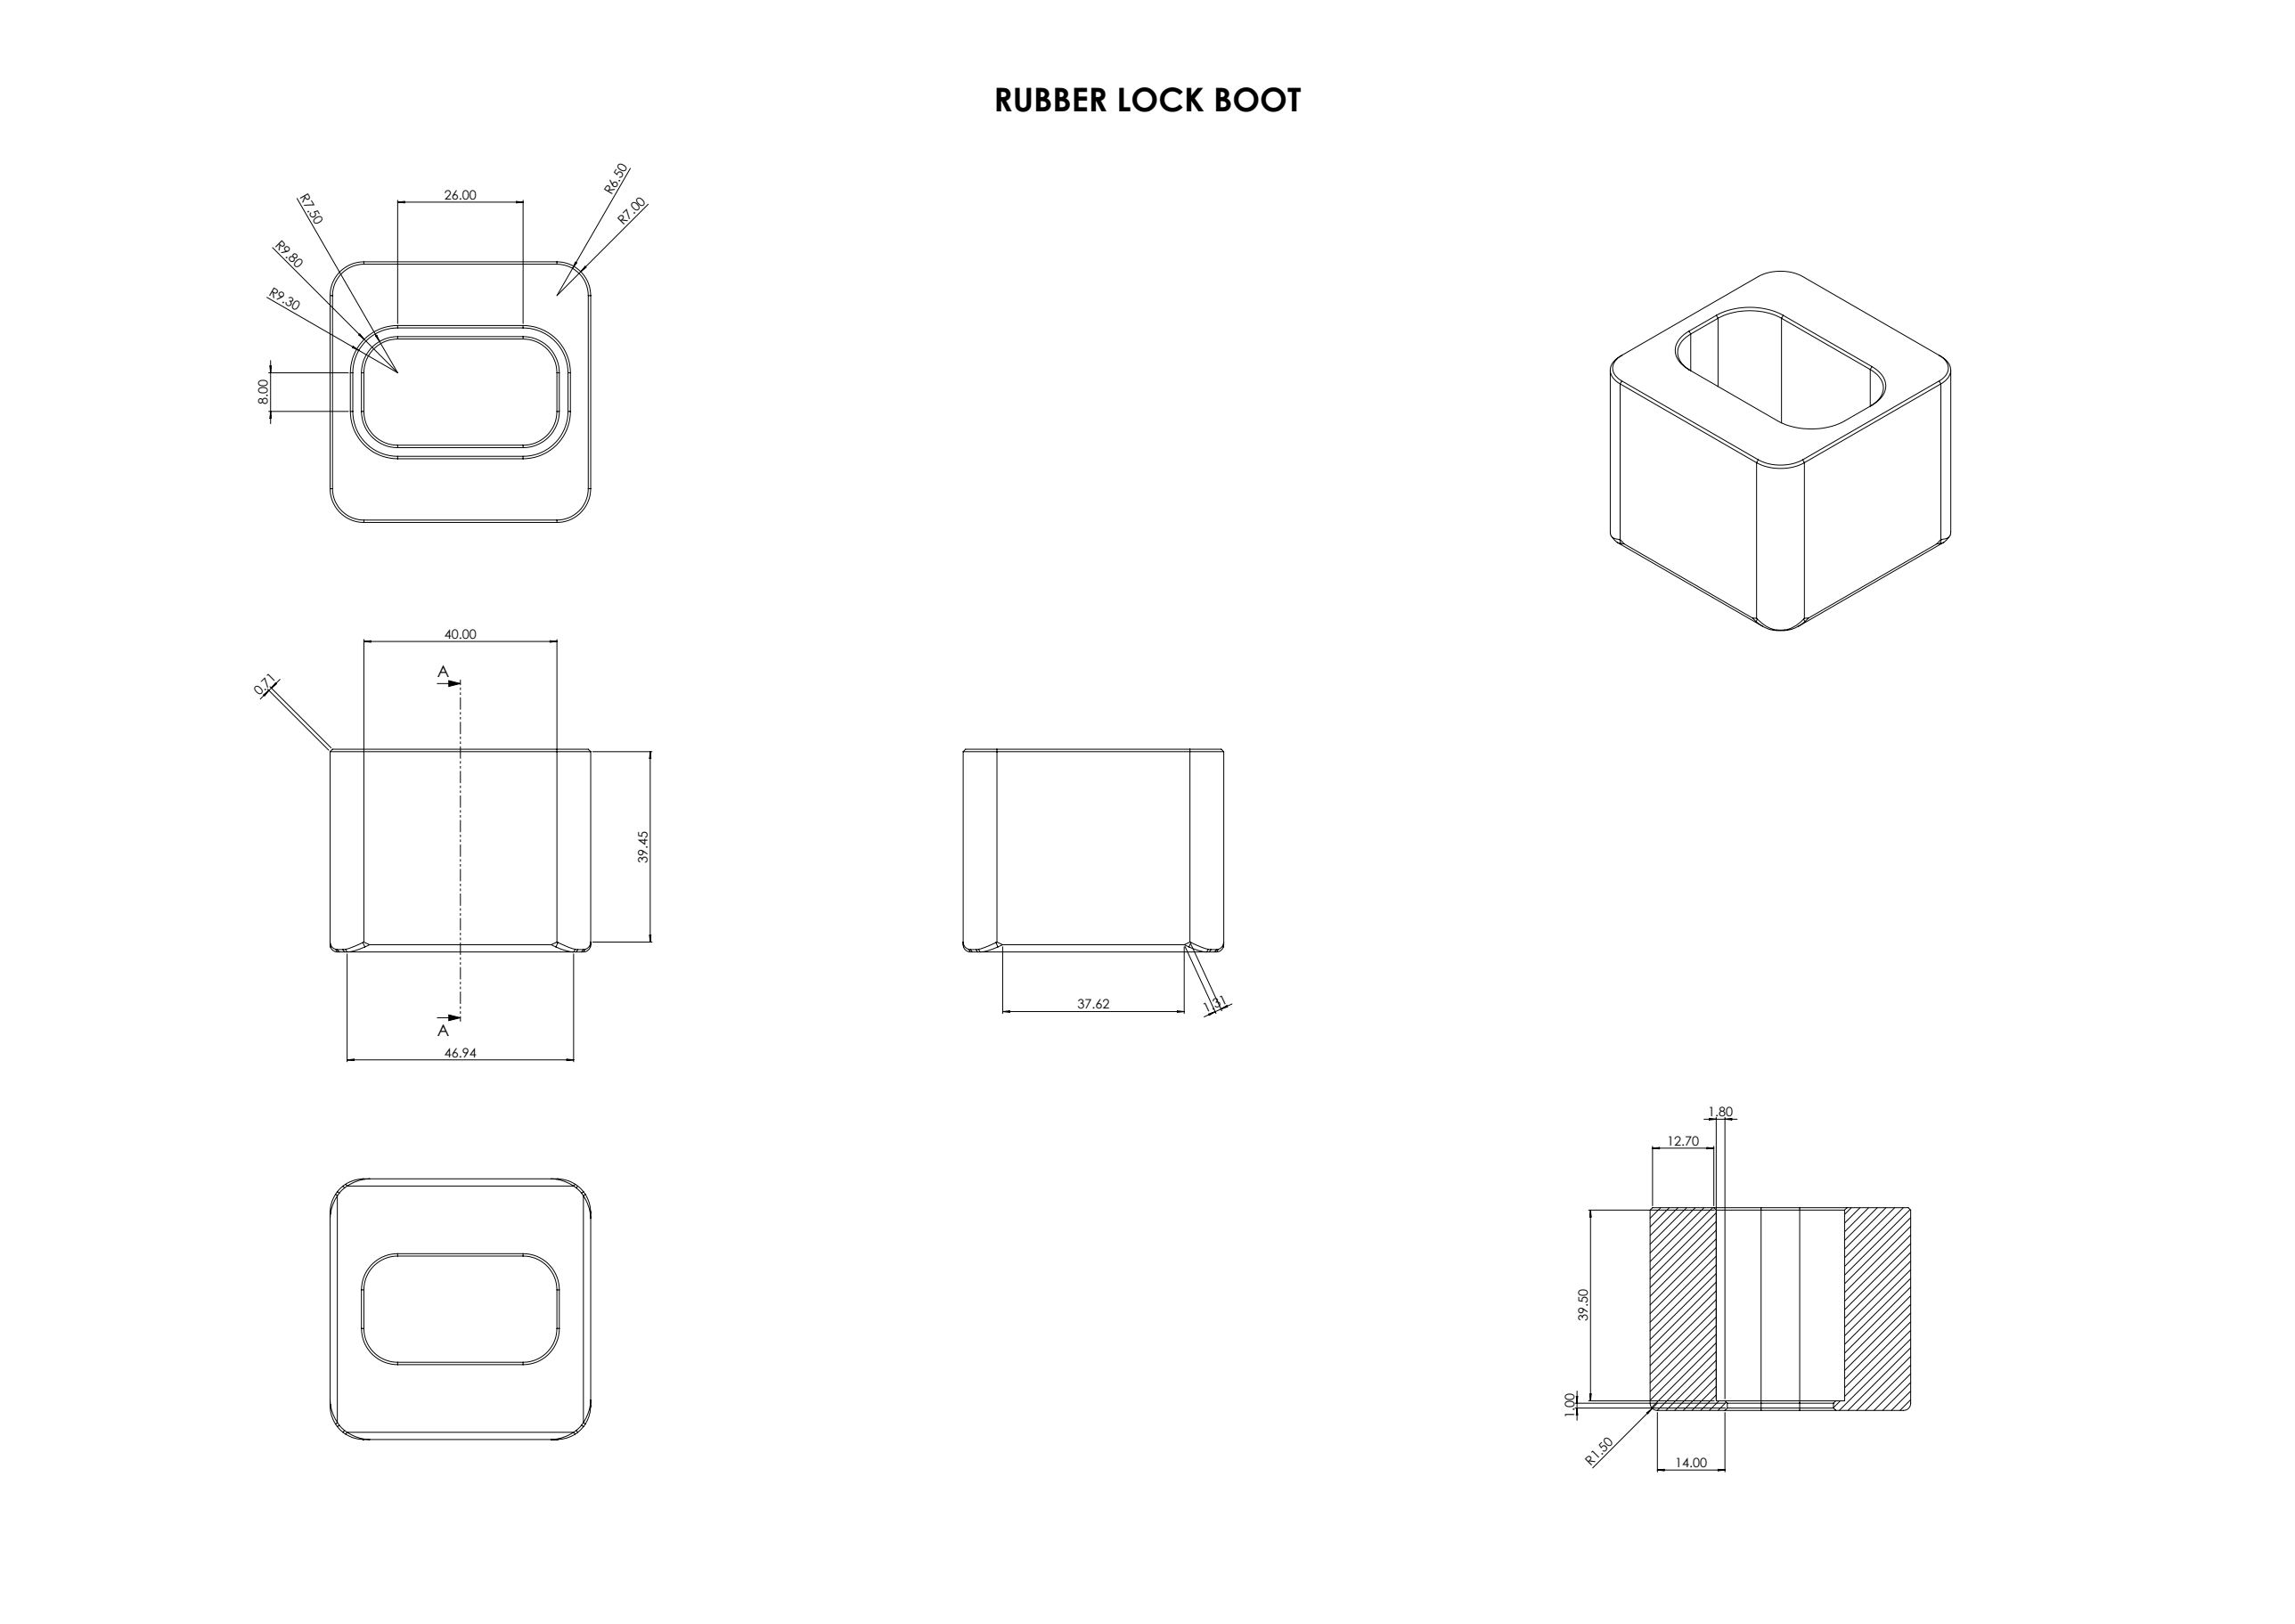
ISO-10303-21;
HEADER;
/* Generated by software containing ST-Developer
 * from STEP Tools, Inc. (www.steptools.com) 
 */

FILE_DESCRIPTION(
/* description */ (''),
/* implementation_level */ '2;1');

FILE_NAME(
/* name */ '13_Rubber_Lock_Boot.step',
/* time_stamp */ '2026-10-25T01:30:15-07:00',
/* author */ (''),
/* organization */ (''),
/* preprocessor_version */ 'ST-DEVELOPER v20.2',
/* originating_system */ 'Autodesk Translation Framework v15.15.0.0',
/* authorisation */ '');

FILE_SCHEMA (('AUTOMOTIVE_DESIGN { 1 0 10303 214 3 1 1 }'));
ENDSEC;

DATA;
#10=MECHANICAL_DESIGN_GEOMETRIC_PRESENTATION_REPRESENTATION('',(#574),#32309);
#296=B_SPLINE_CURVE_WITH_KNOTS('',3,(#27048,#27049,#27050,#27051,#27052,
#27053,#27054,#27055,#27056,#27057,#27058,#27059,#27060,#27061,#27062,#27063,
#27064,#27065,#27066,#27067,#27068,#27069,#27070,#27071,#27072,#27073,#27074,
#27075,#27076,#27077,#27078,#27079,#27080,#27081,#27082,#27083,#27084,#27085,
#27086,#27087,#27088,#27089,#27090,#27091,#27092,#27093,#27094,#27095,#27096,
#27097,#27098,#27099,#27100,#27101,#27102,#27103,#27104,#27105,#27106,#27107,
#27108,#27109,#27110,#27111,#27112,#27113,#27114),.UNSPECIFIED.,.F.,.F.,
(4,3,3,3,3,3,3,3,3,3,3,3,3,3,3,3,3,3,3,3,3,3,4),(0.,0.0372150073459974,
0.0759036440357819,0.116494755002558,0.15971628635105,0.207036887347821,
0.265275351739583,0.328858620274534,0.377066398240659,0.420570421282261,
0.461281571881092,0.50247045159648,0.542638283169258,0.585163636770142,
0.631190064016801,0.685017456026248,0.763763092019686,0.814055107507527,
0.860541330630645,0.901120921336454,0.940124312769201,0.977290078168108,
1.),.UNSPECIFIED.);
#297=B_SPLINE_CURVE_WITH_KNOTS('',3,(#27116,#27117,#27118,#27119,#27120),
 .UNSPECIFIED.,.F.,.F.,(4,1,4),(1.09621611801068,1.29877304187851,1.50132996574633),
 .UNSPECIFIED.);
#298=B_SPLINE_CURVE_WITH_KNOTS('',3,(#27122,#27123,#27124,#27125),
 .UNSPECIFIED.,.F.,.F.,(4,4),(1.02439235355261,1.09621611801068),
 .UNSPECIFIED.);
#299=B_SPLINE_CURVE_WITH_KNOTS('',3,(#27129,#27130,#27131,#27132),
 .UNSPECIFIED.,.F.,.F.,(4,4),(0.396818713712603,0.466059241584687),
 .UNSPECIFIED.);
#300=B_SPLINE_CURVE_WITH_KNOTS('',3,(#27134,#27135,#27136,#27137,#27138,
#27139,#27140),.UNSPECIFIED.,.F.,.F.,(4,2,1,4),(9.99213751786565E-5,0.127637384843918,
0.289146182165162,0.396818713712658),.UNSPECIFIED.);
#301=B_SPLINE_CURVE_WITH_KNOTS('',3,(#27141,#27142,#27143,#27144,#27145,
#27146,#27147,#27148,#27149,#27150,#27151,#27152,#27153,#27154,#27155,#27156,
#27157,#27158,#27159,#27160,#27161,#27162,#27163,#27164,#27165,#27166,#27167,
#27168,#27169,#27170,#27171,#27172,#27173,#27174,#27175,#27176,#27177,#27178,
#27179,#27180,#27181,#27182,#27183,#27184,#27185,#27186,#27187,#27188,#27189,
#27190,#27191,#27192,#27193,#27194,#27195,#27196,#27197,#27198,#27199,#27200,
#27201,#27202,#27203,#27204,#27205,#27206,#27207),.UNSPECIFIED.,.F.,.F.,
(4,3,3,3,3,3,3,3,3,3,3,3,3,3,3,3,3,3,3,3,3,3,4),(0.,0.0372142743249414,
0.0759021060272706,0.116492303751609,0.15971273797737,0.207031854381263,
0.265265992983546,0.328853755149798,0.37706150936917,0.420565256169277,
0.461276052626863,0.50245372219686,0.542621232263039,0.585145966617605,
0.631171144882026,0.684995344588453,0.76374650844134,0.814042029226479,
0.860531521919859,0.901112266515804,0.94011665297404,0.977283203644708,
1.),.UNSPECIFIED.);
#302=B_SPLINE_CURVE_WITH_KNOTS('',3,(#27220,#27221,#27222,#27223,#27224,
#27225,#27226,#27227,#27228,#27229,#27230,#27231,#27232,#27233,#27234,#27235,
#27236,#27237,#27238,#27239,#27240,#27241,#27242,#27243,#27244,#27245,#27246,
#27247,#27248,#27249,#27250,#27251,#27252,#27253,#27254,#27255,#27256,#27257,
#27258,#27259,#27260,#27261,#27262,#27263,#27264,#27265,#27266,#27267,#27268,
#27269,#27270,#27271,#27272,#27273,#27274,#27275,#27276,#27277,#27278,#27279,
#27280,#27281,#27282,#27283,#27284,#27285,#27286),.UNSPECIFIED.,.F.,.F.,
(4,3,3,3,3,3,3,3,3,3,3,3,3,3,3,3,3,3,3,3,3,3,4),(0.,0.0372150196070085,
0.0759036698970674,0.116494796498611,0.15971634697478,0.207036974548953,
0.265275520854355,0.328858695194123,0.377066470534805,0.420570496312742,
0.461281651387635,0.502470683175898,0.542638526520072,0.585163896376155,
0.631190349090315,0.685017798075316,0.763763348556487,0.814055329762754,
0.860541497322065,0.901121082418717,0.94012446955152,0.977290233255848,
1.),.UNSPECIFIED.);
#303=B_SPLINE_CURVE_WITH_KNOTS('',3,(#27288,#27289,#27290,#27291,#27292,
#27293),.UNSPECIFIED.,.F.,.F.,(4,1,1,4),(1.09363288142463,1.20698114379938,
1.26365527498675,1.49035179973623),.UNSPECIFIED.);
#304=B_SPLINE_CURVE_WITH_KNOTS('',3,(#27295,#27296,#27297,#27298),
 .UNSPECIFIED.,.F.,.F.,(4,4),(1.02439235355261,1.09363288142469),
 .UNSPECIFIED.);
#305=B_SPLINE_CURVE_WITH_KNOTS('',3,(#27302,#27303,#27304,#27305),
 .UNSPECIFIED.,.F.,.F.,(4,4),(0.405213665159311,0.477037429617386),
 .UNSPECIFIED.);
#306=B_SPLINE_CURVE_WITH_KNOTS('',3,(#27307,#27308,#27309,#27310,#27311),
 .UNSPECIFIED.,.F.,.F.,(4,1,4),(0.000100096646392837,0.202656880902853,
0.405213665159313),.UNSPECIFIED.);
#307=B_SPLINE_CURVE_WITH_KNOTS('',3,(#27312,#27313,#27314,#27315,#27316,
#27317,#27318,#27319,#27320,#27321,#27322,#27323,#27324,#27325,#27326,#27327,
#27328,#27329,#27330,#27331,#27332,#27333,#27334,#27335,#27336,#27337,#27338,
#27339,#27340,#27341,#27342,#27343,#27344,#27345,#27346,#27347,#27348,#27349,
#27350,#27351,#27352,#27353,#27354,#27355,#27356,#27357,#27358,#27359,#27360,
#27361,#27362,#27363,#27364,#27365,#27366,#27367,#27368,#27369,#27370,#27371,
#27372,#27373,#27374,#27375,#27376,#27377,#27378),.UNSPECIFIED.,.F.,.F.,
(4,3,3,3,3,3,3,3,3,3,3,3,3,3,3,3,3,3,3,3,3,3,4),(0.,0.0372142122738283,
0.0759019766651123,0.116492099285913,0.159712445400096,0.207031446837133,
0.265265278177762,0.328853304622193,0.377061038248202,0.420564750072856,
0.461275507649365,0.502452205884434,0.542619564376986,0.585144107738491,
0.631169015934125,0.684992668379561,0.763744501284671,0.81404021150862,
0.860530158631465,0.901110881237409,0.94011523948485,0.977281743245876,
1.),.UNSPECIFIED.);
#308=B_SPLINE_CURVE_WITH_KNOTS('',3,(#27420,#27421,#27422,#27423,#27424,
#27425,#27426,#27427,#27428,#27429,#27430,#27431,#27432,#27433,#27434,#27435,
#27436,#27437,#27438,#27439,#27440,#27441,#27442,#27443,#27444,#27445,#27446,
#27447,#27448,#27449,#27450,#27451,#27452,#27453,#27454,#27455,#27456,#27457,
#27458,#27459,#27460,#27461,#27462,#27463,#27464,#27465,#27466,#27467,#27468,
#27469,#27470,#27471,#27472,#27473,#27474,#27475,#27476,#27477,#27478,#27479,
#27480,#27481,#27482,#27483,#27484,#27485,#27486,#27487,#27488,#27489,#27490,
#27491,#27492,#27493,#27494,#27495,#27496,#27497,#27498,#27499,#27500,#27501,
#27502,#27503,#27504,#27505,#27506,#27507,#27508,#27509,#27510,#27511,#27512,
#27513,#27514,#27515,#27516),.UNSPECIFIED.,.F.,.F.,(4,3,3,3,3,3,3,3,3,3,
3,3,3,3,3,3,3,3,3,3,3,3,3,3,3,3,3,3,3,3,3,3,4),(0.,0.0249561576389582,0.0505230689649538,
0.0768014946929841,0.103927702815189,0.132729761515055,0.163050828032849,
0.195526914275497,0.231526666456084,0.275596223262613,0.320871459308699,
0.357021183774404,0.38928558844534,0.419345587098888,0.447888984260675,
0.475288232374118,0.503212894511638,0.530052590323374,0.557847043091744,
0.587565866489206,0.619084976767266,0.653310159114776,0.692899272183232,
0.744530806263077,0.780991793284318,0.81370690045686,0.84424865112698,0.87328209994709,
0.901172514215133,0.927739555510914,0.953706026754902,0.978856478652302,
1.),.UNSPECIFIED.);
#309=B_SPLINE_CURVE_WITH_KNOTS('',3,(#27518,#27519,#27520,#27521),
 .UNSPECIFIED.,.F.,.F.,(4,4),(-1.,0.),.UNSPECIFIED.);
#310=B_SPLINE_CURVE_WITH_KNOTS('',3,(#27522,#27523,#27524,#27525,#27526,
#27527,#27528,#27529,#27530,#27531,#27532,#27533,#27534,#27535,#27536,#27537,
#27538,#27539,#27540,#27541,#27542,#27543,#27544,#27545,#27546,#27547,#27548,
#27549,#27550,#27551,#27552,#27553,#27554,#27555,#27556,#27557,#27558,#27559,
#27560,#27561,#27562,#27563,#27564,#27565,#27566,#27567,#27568,#27569,#27570,
#27571,#27572,#27573,#27574,#27575,#27576,#27577,#27578,#27579,#27580,#27581,
#27582,#27583,#27584,#27585,#27586,#27587,#27588),.UNSPECIFIED.,.F.,.F.,
(4,3,3,3,3,3,3,3,3,3,3,3,3,3,3,3,3,3,3,3,3,3,4),(0.,0.037215019607135,0.0759036698970782,
0.116494796498149,0.159716346974602,0.207036974549224,0.265275520853068,
0.328858695193836,0.377066470534692,0.420570496312419,0.461281651387186,
0.502470683172426,0.542638526516054,0.585163896371612,0.631190349085662,
0.685017798068377,0.763763348551283,0.814055329757142,0.860541497317856,
0.901121082414824,0.940124469547107,0.977290233251386,1.),.UNSPECIFIED.);
#311=B_SPLINE_CURVE_WITH_KNOTS('',3,(#27631,#27632,#27633,#27634,#27635,
#27636,#27637,#27638,#27639,#27640,#27641,#27642,#27643,#27644,#27645,#27646,
#27647,#27648,#27649,#27650,#27651,#27652,#27653,#27654,#27655,#27656,#27657,
#27658,#27659,#27660,#27661,#27662,#27663,#27664,#27665,#27666,#27667,#27668,
#27669,#27670,#27671,#27672,#27673,#27674,#27675,#27676,#27677,#27678,#27679,
#27680,#27681,#27682,#27683,#27684,#27685,#27686,#27687,#27688,#27689,#27690,
#27691,#27692,#27693,#27694,#27695,#27696,#27697),.UNSPECIFIED.,.F.,.F.,
(4,3,3,3,3,3,3,3,3,3,3,3,3,3,3,3,3,3,3,3,3,3,4),(0.,0.0372142121292241,
0.0759019763640333,0.116492098810497,0.159712444720991,0.207031445894069,
0.265265276534927,0.328853303564281,0.377061037137402,0.420564748877918,
0.461275506361833,0.502452202278194,0.542619560431093,0.585144103359907,
0.631169010935895,0.684992662113913,0.763744496585435,0.814040207302302,
0.860530155476726,0.901110878061003,0.940115236269481,0.977281739945585,
1.),.UNSPECIFIED.);
#312=B_SPLINE_CURVE_WITH_KNOTS('',3,(#27699,#27700,#27701,#27702),
 .UNSPECIFIED.,.F.,.F.,(4,4),(0.,1.),.UNSPECIFIED.);
#313=B_SPLINE_CURVE_WITH_KNOTS('',3,(#27704,#27705,#27706,#27707,#27708,
#27709,#27710,#27711,#27712,#27713,#27714,#27715,#27716,#27717,#27718,#27719,
#27720,#27721,#27722,#27723,#27724,#27725,#27726,#27727,#27728,#27729,#27730,
#27731,#27732,#27733,#27734,#27735,#27736,#27737,#27738,#27739,#27740,#27741,
#27742,#27743,#27744,#27745,#27746,#27747,#27748,#27749,#27750,#27751,#27752,
#27753,#27754,#27755,#27756,#27757,#27758,#27759,#27760,#27761,#27762,#27763,
#27764,#27765,#27766,#27767,#27768,#27769,#27770,#27771,#27772,#27773,#27774,
#27775,#27776,#27777,#27778,#27779,#27780,#27781,#27782,#27783,#27784,#27785,
#27786,#27787,#27788,#27789,#27790,#27791,#27792,#27793,#27794,#27795,#27796,
#27797,#27798,#27799,#27800),.UNSPECIFIED.,.F.,.F.,(4,3,3,3,3,3,3,3,3,3,
3,3,3,3,3,3,3,3,3,3,3,3,3,3,3,3,3,3,3,3,3,3,4),(0.,0.0249709672790016,0.0505536024514495,
0.0768489351040166,0.103993630089062,0.132817340140775,0.163164016125442,
0.195672955688052,0.231723181390253,0.276005254460143,0.321254926056384,
0.357363044451917,0.389612545656904,0.419666623911194,0.448208487868328,
0.475608730563432,0.503750970182619,0.530595750607696,0.558398676707341,
0.58813364847834,0.619679816365933,0.653955102605481,0.693711324455342,
0.744658928774623,0.781071741936943,0.813756877135301,0.844275170967022,
0.873288582738427,0.901161117024878,0.927712121392446,0.953663439792987,
0.97879939830999,1.),.UNSPECIFIED.);
#314=B_SPLINE_CURVE_WITH_KNOTS('',3,(#27823,#27824,#27825,#27826,#27827),
 .UNSPECIFIED.,.F.,.F.,(4,1,4),(0.000100096646392838,0.202656880902853,
0.405213665159313),.UNSPECIFIED.);
#315=B_SPLINE_CURVE_WITH_KNOTS('',3,(#27830,#27831,#27832,#27833,#27834),
 .UNSPECIFIED.,.F.,.F.,(4,1,4),(-0.405213665159313,-0.202656880902853,-0.000100096646392838),
 .UNSPECIFIED.);
#316=B_SPLINE_CURVE_WITH_KNOTS('',3,(#27860,#27861,#27862,#27863),
 .UNSPECIFIED.,.F.,.F.,(4,4),(-0.477037429617388,-0.405213665159311),
 .UNSPECIFIED.);
#317=B_SPLINE_CURVE_WITH_KNOTS('',3,(#27864,#27865,#27866,#27867),
 .UNSPECIFIED.,.F.,.F.,(4,4),(0.405213665159311,0.477037429617388),
 .UNSPECIFIED.);
#318=B_SPLINE_CURVE_WITH_KNOTS('',3,(#27901,#27902,#27903,#27904,#27905,
#27906,#27907,#27908),.UNSPECIFIED.,.F.,.F.,(4,2,2,4),(-1.49035179973623,
-1.36281421029337,-1.23517682544946,-1.09363288142463),.UNSPECIFIED.);
#319=B_SPLINE_CURVE_WITH_KNOTS('',3,(#27911,#27912,#27913,#27914,#27915,
#27916,#27917,#27918),.UNSPECIFIED.,.F.,.F.,(4,2,2,4),(1.09363288142463,
1.23517682544946,1.36281421029337,1.49035179973623),.UNSPECIFIED.);
#320=B_SPLINE_CURVE_WITH_KNOTS('',3,(#27935,#27936,#27937,#27938),
 .UNSPECIFIED.,.F.,.F.,(4,4),(-1.09363288142469,-1.02439235355261),
 .UNSPECIFIED.);
#321=B_SPLINE_CURVE_WITH_KNOTS('',3,(#27939,#27940,#27941,#27942),
 .UNSPECIFIED.,.F.,.F.,(4,4),(1.02439235355261,1.09363288142469),
 .UNSPECIFIED.);
#322=B_SPLINE_CURVE_WITH_KNOTS('',3,(#27945,#27946,#27947,#27948,#27949,
#27950,#27951,#27952,#27953,#27954,#27955,#27956,#27957,#27958,#27959,#27960,
#27961,#27962,#27963,#27964,#27965,#27966,#27967,#27968,#27969,#27970,#27971,
#27972,#27973,#27974,#27975,#27976,#27977,#27978,#27979,#27980,#27981,#27982,
#27983,#27984,#27985,#27986,#27987,#27988,#27989,#27990,#27991,#27992,#27993,
#27994,#27995,#27996,#27997,#27998,#27999,#28000,#28001,#28002,#28003,#28004,
#28005,#28006,#28007,#28008,#28009,#28010,#28011,#28012,#28013,#28014,#28015,
#28016,#28017,#28018,#28019,#28020,#28021,#28022,#28023,#28024,#28025,#28026,
#28027,#28028,#28029,#28030,#28031,#28032,#28033,#28034,#28035,#28036,#28037,
#28038,#28039,#28040,#28041),.UNSPECIFIED.,.F.,.F.,(4,3,3,3,3,3,3,3,3,3,
3,3,3,3,3,3,3,3,3,3,3,3,3,3,3,3,3,3,3,3,3,3,4),(0.,0.0249709948250819,0.0505536593533966,
0.0768490236852142,0.10399375345847,0.132817504688352,0.163164229887591,
0.195673233277454,0.231723557259323,0.276005984111853,0.321255610104862,
0.357363640101273,0.389613108945727,0.419667173118957,0.448209031765858,
0.475609274173033,0.503751910718119,0.530596724096154,0.558399690027093,
0.588134716371141,0.619680960018544,0.653956366554597,0.693712941226904,
0.744659534140973,0.781072281842521,0.81375738602271,0.844275660836252,
0.873289059550228,0.901161584288134,0.927712584049702,0.953663898808582,
0.978799857569016,1.),.UNSPECIFIED.);
#323=B_SPLINE_CURVE_WITH_KNOTS('',3,(#28043,#28044,#28045,#28046,#28047,
#28048,#28049),.UNSPECIFIED.,.F.,.F.,(4,1,2,4),(-0.396818713712658,-0.289146182165162,
-0.127637384843918,-9.99213751786565E-5),.UNSPECIFIED.);
#324=B_SPLINE_CURVE_WITH_KNOTS('',3,(#28095,#28096,#28097,#28098,#28099,
#28100,#28101,#28102,#28103,#28104,#28105,#28106,#28107,#28108,#28109,#28110,
#28111,#28112,#28113,#28114,#28115,#28116,#28117,#28118,#28119,#28120,#28121,
#28122,#28123,#28124,#28125,#28126,#28127,#28128,#28129,#28130,#28131,#28132,
#28133,#28134,#28135,#28136,#28137,#28138,#28139,#28140,#28141,#28142,#28143,
#28144,#28145,#28146,#28147,#28148,#28149,#28150,#28151,#28152,#28153,#28154,
#28155,#28156,#28157,#28158,#28159,#28160,#28161,#28162,#28163,#28164,#28165,
#28166,#28167,#28168,#28169,#28170,#28171,#28172,#28173,#28174,#28175,#28176,
#28177,#28178,#28179,#28180,#28181,#28182,#28183,#28184,#28185,#28186,#28187,
#28188,#28189,#28190,#28191),.UNSPECIFIED.,.F.,.F.,(4,3,3,3,3,3,3,3,3,3,
3,3,3,3,3,3,3,3,3,3,3,3,3,3,3,3,3,3,3,3,3,3,4),(0.,0.0249561607551759,0.0505230751945413,
0.0768015040119749,0.103927715157316,0.13272977655757,0.163050845426121,
0.195526933356038,0.231526685629517,0.275596237711758,0.320871472854773,
0.357021212133758,0.389285626160042,0.419345632279732,0.447889035910775,
0.475288289852361,0.503212993519124,0.530052682547603,0.557847129410532,
0.587565949393601,0.619085059687446,0.653310249780398,0.692899411004627,
0.744530685907878,0.780991641273838,0.813706725614835,0.844248457013025,
0.873281888573613,0.90117228690679,0.927739312487755,0.953705768715376,
0.978856204742226,1.),.UNSPECIFIED.);
#325=B_SPLINE_CURVE_WITH_KNOTS('',3,(#28193,#28194,#28195,#28196),
 .UNSPECIFIED.,.F.,.F.,(4,4),(-1.,0.),.UNSPECIFIED.);
#326=B_SPLINE_CURVE_WITH_KNOTS('',3,(#28198,#28199,#28200,#28201,#28202,
#28203,#28204,#28205,#28206,#28207,#28208,#28209,#28210,#28211,#28212,#28213,
#28214,#28215,#28216,#28217,#28218,#28219,#28220,#28221,#28222,#28223,#28224,
#28225,#28226,#28227,#28228,#28229,#28230,#28231,#28232,#28233,#28234,#28235,
#28236,#28237,#28238,#28239,#28240,#28241,#28242,#28243,#28244,#28245,#28246,
#28247,#28248,#28249,#28250,#28251,#28252,#28253,#28254,#28255,#28256,#28257,
#28258,#28259,#28260,#28261,#28262,#28263,#28264),.UNSPECIFIED.,.F.,.F.,
(4,3,3,3,3,3,3,3,3,3,3,3,3,3,3,3,3,3,3,3,3,3,4),(0.,0.0372150073460308,
0.075903644036051,0.116494755002737,0.159716286351032,0.207036887346632,
0.265275351737657,0.328858620272782,0.377066398239113,0.420570421280702,
0.461281571879719,0.502470451594025,0.542638283166554,0.585163636766946,
0.631190064013865,0.685017456021953,0.763763092016465,0.814055107505727,
0.860541330629295,0.901120921335073,0.94012431276777,0.977290078166758,
1.),.UNSPECIFIED.);
#327=B_SPLINE_CURVE_WITH_KNOTS('',3,(#28308,#28309,#28310,#28311,#28312,
#28313,#28314,#28315,#28316,#28317,#28318,#28319,#28320,#28321,#28322,#28323,
#28324,#28325,#28326,#28327,#28328,#28329,#28330,#28331,#28332,#28333,#28334,
#28335,#28336,#28337,#28338,#28339,#28340,#28341,#28342,#28343,#28344,#28345,
#28346,#28347,#28348,#28349,#28350,#28351,#28352,#28353,#28354,#28355,#28356,
#28357,#28358,#28359,#28360,#28361,#28362,#28363,#28364,#28365,#28366,#28367,
#28368,#28369,#28370,#28371,#28372,#28373,#28374),.UNSPECIFIED.,.F.,.F.,
(4,3,3,3,3,3,3,3,3,3,3,3,3,3,3,3,3,3,3,3,3,3,4),(0.,0.0372142743247427,
0.0759021060270489,0.116492303751548,0.15971273797765,0.207031854381748,
0.26526599298503,0.328853755151349,0.377061509370842,0.420565256170683,
0.461276052627892,0.502453722200266,0.542621232267039,0.585145966622121,
0.631171144887316,0.684995344592088,0.763746508444066,0.814042029230295,
0.860531521922721,0.901112266518215,0.940116652976414,0.977283203647236,
1.),.UNSPECIFIED.);
#328=B_SPLINE_CURVE_WITH_KNOTS('',3,(#28376,#28377,#28378,#28379),
 .UNSPECIFIED.,.F.,.F.,(4,4),(0.,1.),.UNSPECIFIED.);
#329=B_SPLINE_CURVE_WITH_KNOTS('',3,(#28381,#28382,#28383,#28384,#28385,
#28386,#28387,#28388,#28389,#28390,#28391,#28392,#28393,#28394,#28395,#28396,
#28397,#28398,#28399,#28400,#28401,#28402,#28403,#28404,#28405,#28406,#28407,
#28408,#28409,#28410,#28411,#28412,#28413,#28414,#28415,#28416,#28417,#28418,
#28419,#28420,#28421,#28422,#28423,#28424,#28425,#28426,#28427,#28428,#28429,
#28430,#28431,#28432,#28433,#28434,#28435,#28436,#28437,#28438,#28439,#28440,
#28441,#28442,#28443,#28444,#28445,#28446,#28447,#28448,#28449,#28450,#28451,
#28452,#28453,#28454,#28455,#28456,#28457,#28458,#28459,#28460,#28461,#28462,
#28463,#28464,#28465,#28466,#28467,#28468,#28469,#28470,#28471,#28472,#28473,
#28474,#28475,#28476,#28477),.UNSPECIFIED.,.F.,.F.,(4,3,3,3,3,3,3,3,3,3,
3,3,3,3,3,3,3,3,3,3,3,3,3,3,3,3,3,3,3,3,3,3,4),(0.,0.024970994825275,0.0505536593526047,
0.0768490236835355,0.103993753457102,0.132817504687059,0.163164229886278,
0.195673233276151,0.231723557257424,0.27600598410841,0.321255610101634,
0.357363640098368,0.389613108942904,0.419667173116849,0.448209031763796,
0.475609274170904,0.503751910715254,0.5305967240942,0.558399690026767,0.588134716370664,
0.619680960018106,0.653956366554247,0.69371294122632,0.744659534141732,
0.781072281843131,0.813757386023587,0.844275660837523,0.873289059551439,
0.901161584289068,0.927712584050538,0.953663898809603,0.978799857570089,
1.),.UNSPECIFIED.);
#330=B_SPLINE_CURVE_WITH_KNOTS('',3,(#28512,#28513,#28514,#28515,#28516,
#28517,#28518,#28519),.UNSPECIFIED.,.F.,.F.,(4,2,2,4),(9.99213751786348E-5,
0.127637384843918,0.255274769687837,0.396818713712658),.UNSPECIFIED.);
#331=B_SPLINE_CURVE_WITH_KNOTS('',3,(#28522,#28523,#28524,#28525,#28526,
#28527,#28528,#28529),.UNSPECIFIED.,.F.,.F.,(4,2,2,4),(-0.396818713712658,
-0.255274769687837,-0.127637384843918,-9.99213751786348E-5),
 .UNSPECIFIED.);
#332=B_SPLINE_CURVE_WITH_KNOTS('',3,(#28555,#28556,#28557,#28558),
 .UNSPECIFIED.,.F.,.F.,(4,4),(-0.466059241584687,-0.396818713712602),
 .UNSPECIFIED.);
#333=B_SPLINE_CURVE_WITH_KNOTS('',3,(#28559,#28560,#28561,#28562),
 .UNSPECIFIED.,.F.,.F.,(4,4),(0.396818713712602,0.466059241584687),
 .UNSPECIFIED.);
#334=B_SPLINE_CURVE_WITH_KNOTS('',3,(#28584,#28585,#28586,#28587,#28588),
 .UNSPECIFIED.,.F.,.F.,(4,1,4),(-1.50125809047561,-1.29870116660779,-1.09614424273996),
 .UNSPECIFIED.);
#335=B_SPLINE_CURVE_WITH_KNOTS('',3,(#28591,#28592,#28593,#28594,#28595),
 .UNSPECIFIED.,.F.,.F.,(4,1,4),(1.09614424273996,1.29870116660779,1.50125809047561),
 .UNSPECIFIED.);
#336=B_SPLINE_CURVE_WITH_KNOTS('',3,(#28612,#28613,#28614,#28615),
 .UNSPECIFIED.,.F.,.F.,(4,4),(-1.09614424273996,-1.02432047828189),
 .UNSPECIFIED.);
#337=B_SPLINE_CURVE_WITH_KNOTS('',3,(#28616,#28617,#28618,#28619),
 .UNSPECIFIED.,.F.,.F.,(4,4),(1.02432047828189,1.09614424273996),
 .UNSPECIFIED.);
#338=B_SPLINE_CURVE_WITH_KNOTS('',3,(#28668,#28669,#28670,#28671),
 .UNSPECIFIED.,.F.,.F.,(4,4),(-0.466059241584687,-0.396818713712603),
 .UNSPECIFIED.);
#339=B_SPLINE_CURVE_WITH_KNOTS('',3,(#28675,#28676,#28677,#28678),
 .UNSPECIFIED.,.F.,.F.,(4,4),(-1.09621611801068,-1.02439235355261),
 .UNSPECIFIED.);
#340=B_SPLINE_CURVE_WITH_KNOTS('',3,(#28682,#28683,#28684,#28685),
 .UNSPECIFIED.,.F.,.F.,(4,4),(-0.477037429617386,-0.405213665159311),
 .UNSPECIFIED.);
#341=B_SPLINE_CURVE_WITH_KNOTS('',3,(#28689,#28690,#28691,#28692),
 .UNSPECIFIED.,.F.,.F.,(4,4),(-1.09363288142469,-1.02439235355261),
 .UNSPECIFIED.);
#342=B_SPLINE_CURVE_WITH_KNOTS('',3,(#28735,#28736,#28737,#28738,#28739,
#28740,#28741,#28742,#28743,#28744,#28745,#28746,#28747,#28748,#28749,#28750,
#28751,#28752,#28753,#28754,#28755,#28756,#28757,#28758,#28759,#28760,#28761,
#28762,#28763,#28764,#28765,#28766,#28767,#28768,#28769,#28770,#28771,#28772,
#28773,#28774,#28775,#28776,#28777,#28778,#28779,#28780,#28781,#28782,#28783,
#28784,#28785,#28786,#28787,#28788,#28789,#28790,#28791,#28792,#28793,#28794,
#28795,#28796,#28797,#28798,#28799,#28800,#28801,#28802,#28803,#28804,#28805,
#28806,#28807,#28808,#28809,#28810,#28811,#28812,#28813,#28814,#28815,#28816,
#28817,#28818,#28819,#28820,#28821,#28822,#28823,#28824,#28825,#28826,#28827,
#28828,#28829,#28830,#28831),.UNSPECIFIED.,.F.,.F.,(4,3,3,3,3,3,3,3,3,3,
3,3,3,3,3,3,3,3,3,3,3,3,3,3,3,3,3,3,3,3,3,3,4),(0.,0.0249561607552664,0.0505230751945348,
0.0768015040119973,0.103927715157151,0.132729776557401,0.163050845425953,
0.195526933355796,0.231526685628984,0.275596237711111,0.320871472854167,
0.357021212132904,0.389285626159344,0.419345632279235,0.447889035910456,
0.475288289851987,0.503212993518741,0.530052682547321,0.557847129410434,
0.587565949393458,0.619085059687253,0.653310249780217,0.69289941100446,
0.744530685907743,0.780991641273769,0.813706725614636,0.844248457012843,
0.873281888573462,0.901172286906684,0.927739312487747,0.95370576871536,
0.978856204742182,1.),.UNSPECIFIED.);
#343=B_SPLINE_CURVE_WITH_KNOTS('',3,(#28832,#28833,#28834,#28835),
 .UNSPECIFIED.,.F.,.F.,(4,4),(-1.,0.),.UNSPECIFIED.);
#344=B_SPLINE_CURVE_WITH_KNOTS('',3,(#28876,#28877,#28878,#28879),
 .UNSPECIFIED.,.F.,.F.,(4,4),(0.,1.),.UNSPECIFIED.);
#345=B_SPLINE_CURVE_WITH_KNOTS('',3,(#28948,#28949,#28950,#28951,#28952),
 .UNSPECIFIED.,.F.,.F.,(4,1,4),(-1.50132996574633,-1.29877304187851,-1.09621611801068),
 .UNSPECIFIED.);
#346=B_SPLINE_CURVE_WITH_KNOTS('',3,(#28972,#28973,#28974,#28975,#28976,
#28977,#28978,#28979,#28980,#28981,#28982,#28983,#28984,#28985,#28986,#28987,
#28988,#28989,#28990,#28991,#28992,#28993,#28994,#28995,#28996,#28997,#28998,
#28999,#29000,#29001,#29002,#29003,#29004,#29005,#29006,#29007,#29008,#29009,
#29010,#29011,#29012,#29013,#29014,#29015,#29016,#29017,#29018,#29019,#29020,
#29021,#29022,#29023,#29024,#29025,#29026,#29027,#29028,#29029,#29030,#29031,
#29032,#29033,#29034,#29035,#29036,#29037,#29038,#29039,#29040,#29041,#29042,
#29043,#29044,#29045,#29046,#29047,#29048,#29049,#29050,#29051,#29052,#29053,
#29054,#29055,#29056,#29057,#29058,#29059,#29060,#29061,#29062,#29063,#29064,
#29065,#29066,#29067,#29068),.UNSPECIFIED.,.F.,.F.,(4,3,3,3,3,3,3,3,3,3,
3,3,3,3,3,3,3,3,3,3,3,3,3,3,3,3,3,3,3,3,3,3,4),(0.,0.0249709672484359,0.0505536023890231,
0.076848935008454,0.103993629960391,0.132817339975555,0.163164015919887,
0.195672955438129,0.231723181102756,0.276005254951893,0.321254926517399,
0.357363044848955,0.389612545990367,0.419666624190472,0.448208488100715,
0.475608730754226,0.503750970445978,0.530595750852095,0.558398676932134,
0.588133648681033,0.619679816541673,0.653955102740443,0.693711324443674,
0.744658928150356,0.781071741349566,0.813756876560073,0.844275170394233,
0.873288582162991,0.90116111644343,0.927712120800645,0.953663439191003,
0.978799397693063,1.),.UNSPECIFIED.);
#347=B_SPLINE_CURVE_WITH_KNOTS('',3,(#29069,#29070,#29071,#29072,#29073),
 .UNSPECIFIED.,.F.,.F.,(4,1,4),(-0.405213665159313,-0.202656880902853,-0.000100096646392837),
 .UNSPECIFIED.);
#348=B_SPLINE_CURVE_WITH_KNOTS('',3,(#29116,#29117,#29118,#29119,#29120,
#29121,#29122,#29123,#29124,#29125,#29126,#29127,#29128,#29129,#29130,#29131,
#29132,#29133,#29134,#29135,#29136,#29137,#29138,#29139,#29140,#29141,#29142,
#29143,#29144,#29145,#29146,#29147,#29148,#29149,#29150,#29151,#29152,#29153,
#29154,#29155,#29156,#29157,#29158,#29159,#29160,#29161,#29162,#29163,#29164,
#29165,#29166,#29167,#29168,#29169,#29170,#29171,#29172,#29173,#29174,#29175,
#29176,#29177,#29178,#29179,#29180,#29181,#29182,#29183,#29184,#29185,#29186,
#29187,#29188,#29189,#29190,#29191,#29192,#29193,#29194,#29195,#29196,#29197,
#29198,#29199,#29200,#29201,#29202,#29203,#29204,#29205,#29206,#29207,#29208,
#29209,#29210,#29211,#29212),.UNSPECIFIED.,.F.,.F.,(4,3,3,3,3,3,3,3,3,3,
3,3,3,3,3,3,3,3,3,3,3,3,3,3,3,3,3,3,3,3,3,3,4),(0.,0.0249561576390629,0.0505230689649775,
0.0768014946930641,0.103927702815194,0.132729761515069,0.163050828032914,
0.195526914275558,0.231526666455973,0.275596223262652,0.320871459308736,
0.357021183774344,0.38928558844556,0.419345587099029,0.447888984260831,
0.475288232374163,0.503212894511872,0.530052590323447,0.557847043091724,
0.587565866489155,0.619084976767197,0.653310159114852,0.692899272183628,
0.744530806262874,0.780991793284097,0.813706900456684,0.844248651126759,
0.873282099946833,0.901172514214929,0.927739555510682,0.953706026754719,
0.9788564786521,1.),.UNSPECIFIED.);
#349=B_SPLINE_CURVE_WITH_KNOTS('',3,(#29213,#29214,#29215,#29216),
 .UNSPECIFIED.,.F.,.F.,(4,4),(-1.,0.),.UNSPECIFIED.);
#350=B_SPLINE_CURVE_WITH_KNOTS('',3,(#29258,#29259,#29260,#29261),
 .UNSPECIFIED.,.F.,.F.,(4,4),(0.,1.),.UNSPECIFIED.);
#351=B_SPLINE_CURVE_WITH_KNOTS('',3,(#29326,#29327,#29328,#29329,#29330,
#29331),.UNSPECIFIED.,.F.,.F.,(4,1,1,4),(-1.49035179973623,-1.26365527498675,
-1.20698114379938,-1.09363288142463),.UNSPECIFIED.);
#487=B_SPLINE_SURFACE_WITH_KNOTS('',3,3,((#27379,#27380,#27381,#27382,#27383,
#27384,#27385,#27386,#27387,#27388),(#27389,#27390,#27391,#27392,#27393,
#27394,#27395,#27396,#27397,#27398),(#27399,#27400,#27401,#27402,#27403,
#27404,#27405,#27406,#27407,#27408),(#27409,#27410,#27411,#27412,#27413,
#27414,#27415,#27416,#27417,#27418)),.UNSPECIFIED.,.F.,.F.,.F.,(4,4),(4,
1,1,1,1,1,1,4),(0.,1.),(0.,0.0714285714285714,0.142857142857143,0.428571428571429,
0.571428571428571,0.857142857142857,0.928571428571429,1.),.UNSPECIFIED.);
#488=B_SPLINE_SURFACE_WITH_KNOTS('',3,3,((#27589,#27590,#27591,#27592,#27593,
#27594,#27595,#27596,#27597,#27598),(#27599,#27600,#27601,#27602,#27603,
#27604,#27605,#27606,#27607,#27608),(#27609,#27610,#27611,#27612,#27613,
#27614,#27615,#27616,#27617,#27618),(#27619,#27620,#27621,#27622,#27623,
#27624,#27625,#27626,#27627,#27628)),.UNSPECIFIED.,.F.,.F.,.F.,(4,4),(4,
1,1,1,1,1,1,4),(0.,1.),(0.,0.0714285714285714,0.142857142857143,0.428571428571429,
0.571428571428571,0.857142857142857,0.928571428571429,1.),.UNSPECIFIED.);
#489=B_SPLINE_SURFACE_WITH_KNOTS('',3,3,((#27802,#27803,#27804,#27805,#27806),
(#27807,#27808,#27809,#27810,#27811),(#27812,#27813,#27814,#27815,#27816),
(#27817,#27818,#27819,#27820,#27821)),.UNSPECIFIED.,.F.,.F.,.F.,(4,4),(4,
1,4),(0.,1.),(0.000100096646392838,0.202656880902853,0.405213665159313),
 .UNSPECIFIED.);
#490=B_SPLINE_SURFACE_WITH_KNOTS('',3,3,((#27844,#27845,#27846,#27847),
(#27848,#27849,#27850,#27851),(#27852,#27853,#27854,#27855),(#27856,#27857,
#27858,#27859)),.UNSPECIFIED.,.F.,.F.,.F.,(4,4),(4,4),(0.,1.),(0.405213665159311,
0.477037429617388),.UNSPECIFIED.);
#491=B_SPLINE_SURFACE_WITH_KNOTS('',3,3,((#27868,#27869,#27870,#27871,#27872,
#27873,#27874,#27875),(#27876,#27877,#27878,#27879,#27880,#27881,#27882,
#27883),(#27884,#27885,#27886,#27887,#27888,#27889,#27890,#27891),(#27892,
#27893,#27894,#27895,#27896,#27897,#27898,#27899)),.UNSPECIFIED.,.F.,.F.,
 .F.,(4,4),(4,2,2,4),(0.,1.),(1.09363288142463,1.23517682544946,1.36281421029337,
1.49035179973623),.UNSPECIFIED.);
#492=B_SPLINE_SURFACE_WITH_KNOTS('',3,3,((#27919,#27920,#27921,#27922),
(#27923,#27924,#27925,#27926),(#27927,#27928,#27929,#27930),(#27931,#27932,
#27933,#27934)),.UNSPECIFIED.,.F.,.F.,.F.,(4,4),(4,4),(0.,1.),(1.02439235355261,
1.09363288142469),.UNSPECIFIED.);
#493=B_SPLINE_SURFACE_WITH_KNOTS('',3,3,((#28053,#28054,#28055,#28056,#28057,
#28058,#28059,#28060,#28061,#28062),(#28063,#28064,#28065,#28066,#28067,
#28068,#28069,#28070,#28071,#28072),(#28073,#28074,#28075,#28076,#28077,
#28078,#28079,#28080,#28081,#28082),(#28083,#28084,#28085,#28086,#28087,
#28088,#28089,#28090,#28091,#28092)),.UNSPECIFIED.,.F.,.F.,.F.,(4,4),(4,
1,1,1,1,1,1,4),(0.,1.),(0.,0.0714285714285714,0.142857142857143,0.428571428571429,
0.571428571428571,0.857142857142857,0.928571428571429,1.),.UNSPECIFIED.);
#494=B_SPLINE_SURFACE_WITH_KNOTS('',3,3,((#28266,#28267,#28268,#28269,#28270,
#28271,#28272,#28273,#28274,#28275),(#28276,#28277,#28278,#28279,#28280,
#28281,#28282,#28283,#28284,#28285),(#28286,#28287,#28288,#28289,#28290,
#28291,#28292,#28293,#28294,#28295),(#28296,#28297,#28298,#28299,#28300,
#28301,#28302,#28303,#28304,#28305)),.UNSPECIFIED.,.F.,.F.,.F.,(4,4),(4,
1,1,1,1,1,1,4),(0.,1.),(0.,0.0714285714285714,0.142857142857143,0.428571428571429,
0.571428571428571,0.857142857142857,0.928571428571429,1.),.UNSPECIFIED.);
#495=B_SPLINE_SURFACE_WITH_KNOTS('',3,3,((#28479,#28480,#28481,#28482,#28483,
#28484,#28485,#28486),(#28487,#28488,#28489,#28490,#28491,#28492,#28493,
#28494),(#28495,#28496,#28497,#28498,#28499,#28500,#28501,#28502),(#28503,
#28504,#28505,#28506,#28507,#28508,#28509,#28510)),.UNSPECIFIED.,.F.,.F.,
 .F.,(4,4),(4,2,2,4),(0.,1.),(9.99213751786348E-5,0.127637384843918,0.255274769687837,
0.396818713712658),.UNSPECIFIED.);
#496=B_SPLINE_SURFACE_WITH_KNOTS('',3,3,((#28539,#28540,#28541,#28542),
(#28543,#28544,#28545,#28546),(#28547,#28548,#28549,#28550),(#28551,#28552,
#28553,#28554)),.UNSPECIFIED.,.F.,.F.,.F.,(4,4),(4,4),(0.,1.),(0.396818713712602,
0.466059241584687),.UNSPECIFIED.);
#497=B_SPLINE_SURFACE_WITH_KNOTS('',3,3,((#28563,#28564,#28565,#28566,#28567),
(#28568,#28569,#28570,#28571,#28572),(#28573,#28574,#28575,#28576,#28577),
(#28578,#28579,#28580,#28581,#28582)),.UNSPECIFIED.,.F.,.F.,.F.,(4,4),(4,
1,4),(0.,1.),(1.09614424273996,1.29870116660779,1.50125809047561),
 .UNSPECIFIED.);
#498=B_SPLINE_SURFACE_WITH_KNOTS('',3,3,((#28596,#28597,#28598,#28599),
(#28600,#28601,#28602,#28603),(#28604,#28605,#28606,#28607),(#28608,#28609,
#28610,#28611)),.UNSPECIFIED.,.F.,.F.,.F.,(4,4),(4,4),(0.,1.),(1.02432047828189,
1.09614424273996),.UNSPECIFIED.);
#499=B_SPLINE_SURFACE_WITH_KNOTS('',3,3,((#28694,#28695,#28696,#28697,#28698,
#28699,#28700,#28701,#28702,#28703),(#28704,#28705,#28706,#28707,#28708,
#28709,#28710,#28711,#28712,#28713),(#28714,#28715,#28716,#28717,#28718,
#28719,#28720,#28721,#28722,#28723),(#28724,#28725,#28726,#28727,#28728,
#28729,#28730,#28731,#28732,#28733)),.UNSPECIFIED.,.F.,.F.,.F.,(4,4),(4,
1,1,1,1,1,1,4),(0.,1.),(0.,0.0714285714285714,0.142857142857143,0.428571428571429,
0.571428571428571,0.857142857142857,0.928571428571429,1.),.UNSPECIFIED.);
#500=B_SPLINE_SURFACE_WITH_KNOTS('',3,3,((#28836,#28837,#28838,#28839,#28840,
#28841,#28842,#28843,#28844,#28845),(#28846,#28847,#28848,#28849,#28850,
#28851,#28852,#28853,#28854,#28855),(#28856,#28857,#28858,#28859,#28860,
#28861,#28862,#28863,#28864,#28865),(#28866,#28867,#28868,#28869,#28870,
#28871,#28872,#28873,#28874,#28875)),.UNSPECIFIED.,.F.,.F.,.F.,(4,4),(4,
1,1,1,1,1,1,4),(0.,1.),(0.,0.0714285714285714,0.142857142857143,0.428571428571429,
0.571428571428571,0.857142857142857,0.928571428571429,1.),.UNSPECIFIED.);
#501=B_SPLINE_SURFACE_WITH_KNOTS('',3,3,((#28880,#28881,#28882,#28883,#28884,
#28885,#28886),(#28887,#28888,#28889,#28890,#28891,#28892,#28893),(#28894,
#28895,#28896,#28897,#28898,#28899,#28900),(#28901,#28902,#28903,#28904,
#28905,#28906,#28907)),.UNSPECIFIED.,.F.,.F.,.F.,(4,4),(4,2,1,4),(0.,1.),
(9.99213751786565E-5,0.127637384843918,0.289146182165162,0.396818713712658),
 .UNSPECIFIED.);
#502=B_SPLINE_SURFACE_WITH_KNOTS('',3,3,((#28912,#28913,#28914,#28915),
(#28916,#28917,#28918,#28919),(#28920,#28921,#28922,#28923),(#28924,#28925,
#28926,#28927)),.UNSPECIFIED.,.F.,.F.,.F.,(4,4),(4,4),(0.,1.),(0.396818713712603,
0.466059241584687),.UNSPECIFIED.);
#503=B_SPLINE_SURFACE_WITH_KNOTS('',3,3,((#28928,#28929,#28930,#28931,#28932),
(#28933,#28934,#28935,#28936,#28937),(#28938,#28939,#28940,#28941,#28942),
(#28943,#28944,#28945,#28946,#28947)),.UNSPECIFIED.,.F.,.F.,.F.,(4,4),(4,
1,4),(0.,1.),(1.09621611801068,1.29877304187851,1.50132996574633),
 .UNSPECIFIED.);
#504=B_SPLINE_SURFACE_WITH_KNOTS('',3,3,((#28954,#28955,#28956,#28957),
(#28958,#28959,#28960,#28961),(#28962,#28963,#28964,#28965),(#28966,#28967,
#28968,#28969)),.UNSPECIFIED.,.F.,.F.,.F.,(4,4),(4,4),(0.,1.),(1.02439235355261,
1.09621611801068),.UNSPECIFIED.);
#505=B_SPLINE_SURFACE_WITH_KNOTS('',3,3,((#29074,#29075,#29076,#29077,#29078,
#29079,#29080,#29081,#29082,#29083),(#29084,#29085,#29086,#29087,#29088,
#29089,#29090,#29091,#29092,#29093),(#29094,#29095,#29096,#29097,#29098,
#29099,#29100,#29101,#29102,#29103),(#29104,#29105,#29106,#29107,#29108,
#29109,#29110,#29111,#29112,#29113)),.UNSPECIFIED.,.F.,.F.,.F.,(4,4),(4,
1,1,1,1,1,1,4),(0.,1.),(0.,0.0714285714285714,0.142857142857143,0.428571428571429,
0.571428571428571,0.857142857142857,0.928571428571429,1.),.UNSPECIFIED.);
#506=B_SPLINE_SURFACE_WITH_KNOTS('',3,3,((#29218,#29219,#29220,#29221,#29222,
#29223,#29224,#29225,#29226,#29227),(#29228,#29229,#29230,#29231,#29232,
#29233,#29234,#29235,#29236,#29237),(#29238,#29239,#29240,#29241,#29242,
#29243,#29244,#29245,#29246,#29247),(#29248,#29249,#29250,#29251,#29252,
#29253,#29254,#29255,#29256,#29257)),.UNSPECIFIED.,.F.,.F.,.F.,(4,4),(4,
1,1,1,1,1,1,4),(0.,1.),(0.,0.0714285714285714,0.142857142857143,0.428571428571429,
0.571428571428571,0.857142857142857,0.928571428571429,1.),.UNSPECIFIED.);
#507=B_SPLINE_SURFACE_WITH_KNOTS('',3,3,((#29262,#29263,#29264,#29265,#29266),
(#29267,#29268,#29269,#29270,#29271),(#29272,#29273,#29274,#29275,#29276),
(#29277,#29278,#29279,#29280,#29281)),.UNSPECIFIED.,.F.,.F.,.F.,(4,4),(4,
1,4),(0.,1.),(0.000100096646392837,0.202656880902853,0.405213665159313),
 .UNSPECIFIED.);
#508=B_SPLINE_SURFACE_WITH_KNOTS('',3,3,((#29286,#29287,#29288,#29289),
(#29290,#29291,#29292,#29293),(#29294,#29295,#29296,#29297),(#29298,#29299,
#29300,#29301)),.UNSPECIFIED.,.F.,.F.,.F.,(4,4),(4,4),(0.,1.),(0.405213665159311,
0.477037429617386),.UNSPECIFIED.);
#509=B_SPLINE_SURFACE_WITH_KNOTS('',3,3,((#29302,#29303,#29304,#29305,#29306,
#29307),(#29308,#29309,#29310,#29311,#29312,#29313),(#29314,#29315,#29316,
#29317,#29318,#29319),(#29320,#29321,#29322,#29323,#29324,#29325)),
 .UNSPECIFIED.,.F.,.F.,.F.,(4,4),(4,1,1,4),(0.,1.),(1.09363288142463,1.20698114379938,
1.26365527498675,1.49035179973623),.UNSPECIFIED.);
#510=B_SPLINE_SURFACE_WITH_KNOTS('',3,3,((#29333,#29334,#29335,#29336),
(#29337,#29338,#29339,#29340),(#29341,#29342,#29343,#29344),(#29345,#29346,
#29347,#29348)),.UNSPECIFIED.,.F.,.F.,.F.,(4,4),(4,4),(0.,1.),(1.02439235355261,
1.09363288142469),.UNSPECIFIED.);
#546=SHAPE_REPRESENTATION_RELATIONSHIP('SRR','None',#32373,#560);
#560=ADVANCED_BREP_SHAPE_REPRESENTATION('',(#588),#32306);
#574=STYLED_ITEM('',(#32509),#588);
#588=MANIFOLD_SOLID_BREP('Body1',#13815);
#642=FACE_BOUND('',#2638,.T.);
#643=FACE_BOUND('',#2652,.T.);
#644=FACE_BOUND('',#2693,.T.);
#744=CYLINDRICAL_SURFACE('',#14707,7.00000000000001);
#745=CYLINDRICAL_SURFACE('',#14710,7.);
#746=CYLINDRICAL_SURFACE('',#14735,9.3);
#747=CYLINDRICAL_SURFACE('',#14737,9.3);
#748=CYLINDRICAL_SURFACE('',#14756,7.00000000000001);
#749=CYLINDRICAL_SURFACE('',#14759,7.00000000000001);
#750=CYLINDRICAL_SURFACE('',#14764,1.5);
#751=CYLINDRICAL_SURFACE('',#14765,7.00000000000001);
#752=CYLINDRICAL_SURFACE('',#14769,1.5);
#753=CYLINDRICAL_SURFACE('',#14771,7.00000000000001);
#754=CYLINDRICAL_SURFACE('',#14790,1.5);
#755=CYLINDRICAL_SURFACE('',#14792,1.5);
#756=CYLINDRICAL_SURFACE('',#14795,7.00000000000001);
#757=CYLINDRICAL_SURFACE('',#14797,7.);
#758=CYLINDRICAL_SURFACE('',#14799,9.30000000000001);
#759=CYLINDRICAL_SURFACE('',#14801,9.30000000000001);
#1021=CIRCLE('',#14693,7.5);
#1022=CIRCLE('',#14694,7.);
#1023=CIRCLE('',#14697,7.50000000000001);
#1024=CIRCLE('',#14698,7.00000000000001);
#1025=CIRCLE('',#14701,7.50000000000001);
#1026=CIRCLE('',#14702,7.00000000000001);
#1027=CIRCLE('',#14705,7.5);
#1028=CIRCLE('',#14706,7.);
#1029=CIRCLE('',#14708,7.00000000000001);
#1030=CIRCLE('',#14711,7.);
#1031=CIRCLE('',#14714,9.3);
#1032=CIRCLE('',#14715,9.30000000000001);
#1033=CIRCLE('',#14716,9.30000000000001);
#1034=CIRCLE('',#14717,9.3);
#1035=CIRCLE('',#14719,9.8);
#1036=CIRCLE('',#14720,9.3);
#1037=CIRCLE('',#14723,9.8);
#1038=CIRCLE('',#14724,9.3);
#1039=CIRCLE('',#14727,9.80000000000001);
#1040=CIRCLE('',#14728,9.30000000000001);
#1041=CIRCLE('',#14731,9.80000000000001);
#1042=CIRCLE('',#14732,9.30000000000001);
#1043=CIRCLE('',#14739,6.50000000000001);
#1044=CIRCLE('',#14740,6.50000000000001);
#1045=CIRCLE('',#14741,6.50000000000001);
#1046=CIRCLE('',#14742,6.50000000000001);
#1047=CIRCLE('',#14744,7.00000000000001);
#1048=CIRCLE('',#14747,7.00000000000001);
#1049=CIRCLE('',#14750,7.00000000000001);
#1050=CIRCLE('',#14753,7.00000000000001);
#1051=CIRCLE('',#14757,7.00000000000001);
#1052=CIRCLE('',#14760,7.00000000000001);
#1053=CIRCLE('',#14762,6.50000000000001);
#1054=CIRCLE('',#14763,7.00000000000001);
#1055=CIRCLE('',#14767,6.50000000000001);
#1056=CIRCLE('',#14768,7.00000000000001);
#1057=CIRCLE('',#14773,7.50000000000001);
#1058=CIRCLE('',#14776,7.5);
#1059=CIRCLE('',#14779,7.5);
#1060=CIRCLE('',#14780,7.);
#1061=CIRCLE('',#14783,7.50000000000001);
#1062=CIRCLE('',#14784,7.00000000000001);
#1063=CIRCLE('',#14787,6.50000000000001);
#1064=CIRCLE('',#14788,6.50000000000001);
#1208=CONICAL_SURFACE('',#14692,7.25,0.785398163397452);
#1209=CONICAL_SURFACE('',#14696,7.25000000000001,0.785398163397451);
#1210=CONICAL_SURFACE('',#14700,7.25000000000001,0.785398163397451);
#1211=CONICAL_SURFACE('',#14704,7.25,0.785398163397452);
#1212=CONICAL_SURFACE('',#14718,9.55,0.785398163397451);
#1213=CONICAL_SURFACE('',#14722,9.55,0.785398163397449);
#1214=CONICAL_SURFACE('',#14726,9.55,0.785398163397449);
#1215=CONICAL_SURFACE('',#14730,9.55000000000001,0.785398163397449);
#1216=CONICAL_SURFACE('',#14743,6.75000000000001,0.785398163397449);
#1217=CONICAL_SURFACE('',#14746,6.75000000000001,0.785398163397449);
#1218=CONICAL_SURFACE('',#14749,6.75000000000001,0.785398163397451);
#1219=CONICAL_SURFACE('',#14752,6.75000000000001,0.785398163397449);
#1220=CONICAL_SURFACE('',#14761,6.75000000000001,0.785398163397451);
#1221=CONICAL_SURFACE('',#14766,6.75000000000001,0.785398163397449);
#1222=CONICAL_SURFACE('',#14772,7.25000000000001,0.785398163397451);
#1223=CONICAL_SURFACE('',#14775,7.25,0.785398163397452);
#1224=CONICAL_SURFACE('',#14778,7.25,0.785398163397452);
#1225=CONICAL_SURFACE('',#14782,7.25000000000001,0.785398163397451);
#1226=CONICAL_SURFACE('',#14789,6.75000000000001,0.785398163397449);
#1227=CONICAL_SURFACE('',#14791,6.75000000000001,0.785398163397449);
#1775=FACE_OUTER_BOUND('',#2625,.T.);
#1776=FACE_OUTER_BOUND('',#2626,.T.);
#1777=FACE_OUTER_BOUND('',#2627,.T.);
#1778=FACE_OUTER_BOUND('',#2628,.T.);
#1779=FACE_OUTER_BOUND('',#2629,.T.);
#1780=FACE_OUTER_BOUND('',#2630,.T.);
#1781=FACE_OUTER_BOUND('',#2631,.T.);
#1782=FACE_OUTER_BOUND('',#2632,.T.);
#1783=FACE_OUTER_BOUND('',#2633,.T.);
#1784=FACE_OUTER_BOUND('',#2634,.T.);
#1785=FACE_OUTER_BOUND('',#2635,.T.);
#1786=FACE_OUTER_BOUND('',#2636,.T.);
#1787=FACE_OUTER_BOUND('',#2637,.T.);
#1788=FACE_OUTER_BOUND('',#2639,.T.);
#1789=FACE_OUTER_BOUND('',#2640,.T.);
#1790=FACE_OUTER_BOUND('',#2641,.T.);
#1791=FACE_OUTER_BOUND('',#2642,.T.);
#1792=FACE_OUTER_BOUND('',#2643,.T.);
#1793=FACE_OUTER_BOUND('',#2644,.T.);
#1794=FACE_OUTER_BOUND('',#2645,.T.);
#1795=FACE_OUTER_BOUND('',#2646,.T.);
#1796=FACE_OUTER_BOUND('',#2647,.T.);
#1797=FACE_OUTER_BOUND('',#2648,.T.);
#1798=FACE_OUTER_BOUND('',#2649,.T.);
#1799=FACE_OUTER_BOUND('',#2650,.T.);
#1800=FACE_OUTER_BOUND('',#2651,.T.);
#1801=FACE_OUTER_BOUND('',#2653,.T.);
#1802=FACE_OUTER_BOUND('',#2654,.T.);
#1803=FACE_OUTER_BOUND('',#2655,.T.);
#1804=FACE_OUTER_BOUND('',#2656,.T.);
#1805=FACE_OUTER_BOUND('',#2657,.T.);
#1806=FACE_OUTER_BOUND('',#2658,.T.);
#1807=FACE_OUTER_BOUND('',#2659,.T.);
#1808=FACE_OUTER_BOUND('',#2660,.T.);
#1809=FACE_OUTER_BOUND('',#2661,.T.);
#1810=FACE_OUTER_BOUND('',#2662,.T.);
#1811=FACE_OUTER_BOUND('',#2663,.T.);
#1812=FACE_OUTER_BOUND('',#2664,.T.);
#1813=FACE_OUTER_BOUND('',#2665,.T.);
#1814=FACE_OUTER_BOUND('',#2666,.T.);
#1815=FACE_OUTER_BOUND('',#2667,.T.);
#1816=FACE_OUTER_BOUND('',#2668,.T.);
#1817=FACE_OUTER_BOUND('',#2669,.T.);
#1818=FACE_OUTER_BOUND('',#2670,.T.);
#1819=FACE_OUTER_BOUND('',#2671,.T.);
#1820=FACE_OUTER_BOUND('',#2672,.T.);
#1821=FACE_OUTER_BOUND('',#2673,.T.);
#1822=FACE_OUTER_BOUND('',#2674,.T.);
#1823=FACE_OUTER_BOUND('',#2675,.T.);
#1824=FACE_OUTER_BOUND('',#2676,.T.);
#1825=FACE_OUTER_BOUND('',#2677,.T.);
#1826=FACE_OUTER_BOUND('',#2678,.T.);
#1827=FACE_OUTER_BOUND('',#2679,.T.);
#1828=FACE_OUTER_BOUND('',#2680,.T.);
#1829=FACE_OUTER_BOUND('',#2681,.T.);
#1830=FACE_OUTER_BOUND('',#2682,.T.);
#1831=FACE_OUTER_BOUND('',#2683,.T.);
#1832=FACE_OUTER_BOUND('',#2684,.T.);
#1833=FACE_OUTER_BOUND('',#2685,.T.);
#1834=FACE_OUTER_BOUND('',#2686,.T.);
#1835=FACE_OUTER_BOUND('',#2687,.T.);
#1836=FACE_OUTER_BOUND('',#2688,.T.);
#1837=FACE_OUTER_BOUND('',#2689,.T.);
#1838=FACE_OUTER_BOUND('',#2690,.T.);
#1839=FACE_OUTER_BOUND('',#2691,.T.);
#1840=FACE_OUTER_BOUND('',#2692,.T.);
#1841=FACE_OUTER_BOUND('',#2694,.T.);
#1842=FACE_OUTER_BOUND('',#2695,.T.);
#1843=FACE_OUTER_BOUND('',#2696,.T.);
#1844=FACE_OUTER_BOUND('',#2697,.T.);
#1845=FACE_OUTER_BOUND('',#2698,.T.);
#1846=FACE_OUTER_BOUND('',#2699,.T.);
#1847=FACE_OUTER_BOUND('',#2700,.T.);
#1848=FACE_OUTER_BOUND('',#2701,.T.);
#1849=FACE_OUTER_BOUND('',#2702,.T.);
#1850=FACE_OUTER_BOUND('',#2703,.T.);
#1851=FACE_OUTER_BOUND('',#2704,.T.);
#1852=FACE_OUTER_BOUND('',#2705,.T.);
#1853=FACE_OUTER_BOUND('',#2706,.T.);
#1854=FACE_OUTER_BOUND('',#2707,.T.);
#1855=FACE_OUTER_BOUND('',#2708,.T.);
#1856=FACE_OUTER_BOUND('',#2709,.T.);
#1857=FACE_OUTER_BOUND('',#2710,.T.);
#1858=FACE_OUTER_BOUND('',#2711,.T.);
#1859=FACE_OUTER_BOUND('',#2712,.T.);
#1860=FACE_OUTER_BOUND('',#2713,.T.);
#1861=FACE_OUTER_BOUND('',#2714,.T.);
#1862=FACE_OUTER_BOUND('',#2715,.T.);
#1863=FACE_OUTER_BOUND('',#2716,.T.);
#1864=FACE_OUTER_BOUND('',#2717,.T.);
#1865=FACE_OUTER_BOUND('',#2718,.T.);
#2625=EDGE_LOOP('',(#11251,#11252,#11253,#11254));
#2626=EDGE_LOOP('',(#11255,#11256,#11257,#11258));
#2627=EDGE_LOOP('',(#11259,#11260,#11261,#11262));
#2628=EDGE_LOOP('',(#11263,#11264,#11265,#11266));
#2629=EDGE_LOOP('',(#11267,#11268,#11269,#11270));
#2630=EDGE_LOOP('',(#11271,#11272,#11273,#11274));
#2631=EDGE_LOOP('',(#11275,#11276,#11277,#11278));
#2632=EDGE_LOOP('',(#11279,#11280,#11281,#11282));
#2633=EDGE_LOOP('',(#11283,#11284,#11285,#11286));
#2634=EDGE_LOOP('',(#11287,#11288,#11289,#11290));
#2635=EDGE_LOOP('',(#11291,#11292,#11293,#11294));
#2636=EDGE_LOOP('',(#11295,#11296,#11297,#11298));
#2637=EDGE_LOOP('',(#11299,#11300,#11301,#11302,#11303,#11304,#11305,#11306));
#2638=EDGE_LOOP('',(#11307,#11308,#11309,#11310,#11311,#11312,#11313,#11314));
#2639=EDGE_LOOP('',(#11315,#11316,#11317,#11318));
#2640=EDGE_LOOP('',(#11319,#11320,#11321,#11322));
#2641=EDGE_LOOP('',(#11323,#11324,#11325,#11326));
#2642=EDGE_LOOP('',(#11327,#11328,#11329,#11330));
#2643=EDGE_LOOP('',(#11331,#11332,#11333,#11334));
#2644=EDGE_LOOP('',(#11335,#11336,#11337,#11338));
#2645=EDGE_LOOP('',(#11339,#11340,#11341,#11342));
#2646=EDGE_LOOP('',(#11343,#11344,#11345,#11346));
#2647=EDGE_LOOP('',(#11347,#11348,#11349,#11350));
#2648=EDGE_LOOP('',(#11351,#11352,#11353,#11354));
#2649=EDGE_LOOP('',(#11355,#11356,#11357,#11358));
#2650=EDGE_LOOP('',(#11359,#11360,#11361,#11362));
#2651=EDGE_LOOP('',(#11363,#11364,#11365,#11366,#11367,#11368,#11369,#11370));
#2652=EDGE_LOOP('',(#11371,#11372,#11373,#11374,#11375,#11376,#11377,#11378));
#2653=EDGE_LOOP('',(#11379,#11380,#11381,#11382));
#2654=EDGE_LOOP('',(#11383,#11384,#11385,#11386));
#2655=EDGE_LOOP('',(#11387,#11388,#11389,#11390));
#2656=EDGE_LOOP('',(#11391,#11392,#11393,#11394));
#2657=EDGE_LOOP('',(#11395,#11396,#11397,#11398));
#2658=EDGE_LOOP('',(#11399,#11400,#11401,#11402));
#2659=EDGE_LOOP('',(#11403,#11404,#11405,#11406));
#2660=EDGE_LOOP('',(#11407,#11408,#11409,#11410));
#2661=EDGE_LOOP('',(#11411,#11412,#11413,#11414,#11415,#11416));
#2662=EDGE_LOOP('',(#11417,#11418,#11419,#11420,#11421,#11422,#11423,#11424,
#11425,#11426));
#2663=EDGE_LOOP('',(#11427,#11428,#11429,#11430,#11431,#11432));
#2664=EDGE_LOOP('',(#11433,#11434,#11435,#11436,#11437,#11438,#11439,#11440,
#11441,#11442));
#2665=EDGE_LOOP('',(#11443,#11444,#11445,#11446));
#2666=EDGE_LOOP('',(#11447,#11448,#11449,#11450));
#2667=EDGE_LOOP('',(#11451,#11452,#11453,#11454));
#2668=EDGE_LOOP('',(#11455,#11456,#11457,#11458));
#2669=EDGE_LOOP('',(#11459,#11460,#11461,#11462));
#2670=EDGE_LOOP('',(#11463,#11464,#11465,#11466));
#2671=EDGE_LOOP('',(#11467,#11468,#11469,#11470));
#2672=EDGE_LOOP('',(#11471,#11472,#11473,#11474,#11475,#11476));
#2673=EDGE_LOOP('',(#11477,#11478,#11479,#11480,#11481,#11482,#11483,#11484,
#11485,#11486));
#2674=EDGE_LOOP('',(#11487,#11488,#11489,#11490));
#2675=EDGE_LOOP('',(#11491,#11492,#11493,#11494));
#2676=EDGE_LOOP('',(#11495,#11496,#11497,#11498));
#2677=EDGE_LOOP('',(#11499,#11500,#11501,#11502));
#2678=EDGE_LOOP('',(#11503,#11504,#11505,#11506));
#2679=EDGE_LOOP('',(#11507,#11508,#11509,#11510));
#2680=EDGE_LOOP('',(#11511,#11512,#11513,#11514));
#2681=EDGE_LOOP('',(#11515,#11516,#11517,#11518,#11519,#11520));
#2682=EDGE_LOOP('',(#11521,#11522,#11523,#11524,#11525,#11526));
#2683=EDGE_LOOP('',(#11527,#11528,#11529,#11530,#11531,#11532,#11533,#11534,
#11535,#11536));
#2684=EDGE_LOOP('',(#11537,#11538,#11539,#11540));
#2685=EDGE_LOOP('',(#11541,#11542,#11543,#11544));
#2686=EDGE_LOOP('',(#11545,#11546,#11547,#11548));
#2687=EDGE_LOOP('',(#11549,#11550,#11551,#11552));
#2688=EDGE_LOOP('',(#11553,#11554,#11555,#11556));
#2689=EDGE_LOOP('',(#11557,#11558,#11559,#11560));
#2690=EDGE_LOOP('',(#11561,#11562,#11563,#11564));
#2691=EDGE_LOOP('',(#11565,#11566,#11567,#11568));
#2692=EDGE_LOOP('',(#11569,#11570,#11571,#11572,#11573,#11574,#11575,#11576,
#11577,#11578,#11579,#11580,#11581,#11582,#11583,#11584));
#2693=EDGE_LOOP('',(#11585,#11586,#11587,#11588,#11589,#11590,#11591,#11592));
#2694=EDGE_LOOP('',(#11593,#11594,#11595,#11596));
#2695=EDGE_LOOP('',(#11597,#11598,#11599,#11600));
#2696=EDGE_LOOP('',(#11601,#11602,#11603,#11604));
#2697=EDGE_LOOP('',(#11605,#11606,#11607,#11608));
#2698=EDGE_LOOP('',(#11609,#11610,#11611,#11612));
#2699=EDGE_LOOP('',(#11613,#11614,#11615,#11616));
#2700=EDGE_LOOP('',(#11617,#11618,#11619,#11620));
#2701=EDGE_LOOP('',(#11621,#11622,#11623,#11624,#11625,#11626));
#2702=EDGE_LOOP('',(#11627,#11628,#11629,#11630));
#2703=EDGE_LOOP('',(#11631,#11632,#11633,#11634));
#2704=EDGE_LOOP('',(#11635,#11636,#11637,#11638));
#2705=EDGE_LOOP('',(#11639,#11640,#11641,#11642));
#2706=EDGE_LOOP('',(#11643,#11644,#11645,#11646));
#2707=EDGE_LOOP('',(#11647,#11648,#11649,#11650));
#2708=EDGE_LOOP('',(#11651,#11652,#11653,#11654));
#2709=EDGE_LOOP('',(#11655,#11656,#11657,#11658,#11659,#11660));
#2710=EDGE_LOOP('',(#11661,#11662,#11663,#11664,#11665,#11666));
#2711=EDGE_LOOP('',(#11667,#11668,#11669,#11670));
#2712=EDGE_LOOP('',(#11671,#11672,#11673,#11674));
#2713=EDGE_LOOP('',(#11675,#11676,#11677,#11678));
#2714=EDGE_LOOP('',(#11679,#11680,#11681,#11682));
#2715=EDGE_LOOP('',(#11683,#11684,#11685,#11686));
#2716=EDGE_LOOP('',(#11687,#11688,#11689,#11690));
#2717=EDGE_LOOP('',(#11691,#11692,#11693,#11694));
#2718=EDGE_LOOP('',(#11695,#11696,#11697,#11698));
#3718=LINE('',#26848,#5029);
#3719=LINE('',#26850,#5030);
#3720=LINE('',#26852,#5031);
#3721=LINE('',#26853,#5032);
#3722=LINE('',#26857,#5033);
#3723=LINE('',#26863,#5034);
#3724=LINE('',#26864,#5035);
#3725=LINE('',#26865,#5036);
#3726=LINE('',#26869,#5037);
#3727=LINE('',#26875,#5038);
#3728=LINE('',#26876,#5039);
#3729=LINE('',#26877,#5040);
#3730=LINE('',#26881,#5041);
#3731=LINE('',#26887,#5042);
#3732=LINE('',#26888,#5043);
#3733=LINE('',#26889,#5044);
#3734=LINE('',#26895,#5045);
#3735=LINE('',#26898,#5046);
#3736=LINE('',#26901,#5047);
#3737=LINE('',#26902,#5048);
#3738=LINE('',#26905,#5049);
#3739=LINE('',#26909,#5050);
#3740=LINE('',#26910,#5051);
#3741=LINE('',#26914,#5052);
#3742=LINE('',#26918,#5053);
#3743=LINE('',#26922,#5054);
#3744=LINE('',#26926,#5055);
#3745=LINE('',#26931,#5056);
#3746=LINE('',#26935,#5057);
#3747=LINE('',#26940,#5058);
#3748=LINE('',#26941,#5059);
#3749=LINE('',#26942,#5060);
#3750=LINE('',#26946,#5061);
#3751=LINE('',#26952,#5062);
#3752=LINE('',#26953,#5063);
#3753=LINE('',#26954,#5064);
#3754=LINE('',#26958,#5065);
#3755=LINE('',#26964,#5066);
#3756=LINE('',#26965,#5067);
#3757=LINE('',#26966,#5068);
#3758=LINE('',#26970,#5069);
#3759=LINE('',#26974,#5070);
#3760=LINE('',#26975,#5071);
#3761=LINE('',#26977,#5072);
#3762=LINE('',#26978,#5073);
#3763=LINE('',#26980,#5074);
#3764=LINE('',#26982,#5075);
#3765=LINE('',#26984,#5076);
#3766=LINE('',#26990,#5077);
#3767=LINE('',#26994,#5078);
#3768=LINE('',#26998,#5079);
#3769=LINE('',#27001,#5080);
#3770=LINE('',#27004,#5081);
#3771=LINE('',#27006,#5082);
#3772=LINE('',#27010,#5083);
#3773=LINE('',#27011,#5084);
#3774=LINE('',#27014,#5085);
#3775=LINE('',#27018,#5086);
#3776=LINE('',#27019,#5087);
#3777=LINE('',#27022,#5088);
#3778=LINE('',#27026,#5089);
#3779=LINE('',#27027,#5090);
#3780=LINE('',#27030,#5091);
#3781=LINE('',#27033,#5092);
#3782=LINE('',#27036,#5093);
#3783=LINE('',#27038,#5094);
#3784=LINE('',#27040,#5095);
#3785=LINE('',#27042,#5096);
#3786=LINE('',#27043,#5097);
#3787=LINE('',#27046,#5098);
#3788=LINE('',#27210,#5099);
#3789=LINE('',#27212,#5100);
#3790=LINE('',#27214,#5101);
#3791=LINE('',#27215,#5102);
#3792=LINE('',#27218,#5103);
#3793=LINE('',#27801,#5104);
#3794=LINE('',#27829,#5105);
#3795=LINE('',#27838,#5106);
#3796=LINE('',#27842,#5107);
#3797=LINE('',#27910,#5108);
#3798=LINE('',#28050,#5109);
#3799=LINE('',#28052,#5110);
#3800=LINE('',#28265,#5111);
#3801=LINE('',#28478,#5112);
#3802=LINE('',#28521,#5113);
#3803=LINE('',#28533,#5114);
#3804=LINE('',#28537,#5115);
#3805=LINE('',#28590,#5116);
#3806=LINE('',#28621,#5117);
#3807=LINE('',#28622,#5118);
#3808=LINE('',#28624,#5119);
#3809=LINE('',#28626,#5120);
#3810=LINE('',#28629,#5121);
#3811=LINE('',#28632,#5122);
#3812=LINE('',#28635,#5123);
#3813=LINE('',#28636,#5124);
#3814=LINE('',#28639,#5125);
#3815=LINE('',#28643,#5126);
#3816=LINE('',#28644,#5127);
#3817=LINE('',#28648,#5128);
#3818=LINE('',#28654,#5129);
#3819=LINE('',#28655,#5130);
#3820=LINE('',#28656,#5131);
#3821=LINE('',#28660,#5132);
#3822=LINE('',#28664,#5133);
#3823=LINE('',#28665,#5134);
#3824=LINE('',#28680,#5135);
#3825=LINE('',#28693,#5136);
#3826=LINE('',#28908,#5137);
#3827=LINE('',#28910,#5138);
#3828=LINE('',#28911,#5139);
#3829=LINE('',#28953,#5140);
#3830=LINE('',#29217,#5141);
#3831=LINE('',#29282,#5142);
#3832=LINE('',#29284,#5143);
#3833=LINE('',#29285,#5144);
#3834=LINE('',#29332,#5145);
#3835=LINE('',#29350,#5146);
#3836=LINE('',#29353,#5147);
#3837=LINE('',#29355,#5148);
#3838=LINE('',#29357,#5149);
#3839=LINE('',#29360,#5150);
#3840=LINE('',#29361,#5151);
#3841=LINE('',#29363,#5152);
#5029=VECTOR('',#17264,10.);
#5030=VECTOR('',#17265,10.);
#5031=VECTOR('',#17266,10.);
#5032=VECTOR('',#17267,10.);
#5033=VECTOR('',#17270,10.);
#5034=VECTOR('',#17277,10.);
#5035=VECTOR('',#17278,10.);
#5036=VECTOR('',#17279,10.);
#5037=VECTOR('',#17282,10.);
#5038=VECTOR('',#17289,10.);
#5039=VECTOR('',#17290,10.);
#5040=VECTOR('',#17291,10.);
#5041=VECTOR('',#17294,10.);
#5042=VECTOR('',#17301,10.);
#5043=VECTOR('',#17302,10.);
#5044=VECTOR('',#17303,10.);
#5045=VECTOR('',#17312,10.);
#5046=VECTOR('',#17315,10.);
#5047=VECTOR('',#17318,10.);
#5048=VECTOR('',#17319,10.);
#5049=VECTOR('',#17322,10.);
#5050=VECTOR('',#17327,10.);
#5051=VECTOR('',#17328,10.);
#5052=VECTOR('',#17331,10.);
#5053=VECTOR('',#17334,10.);
#5054=VECTOR('',#17337,10.);
#5055=VECTOR('',#17340,10.);
#5056=VECTOR('',#17345,10.);
#5057=VECTOR('',#17348,10.);
#5058=VECTOR('',#17353,10.);
#5059=VECTOR('',#17354,10.);
#5060=VECTOR('',#17355,10.);
#5061=VECTOR('',#17358,10.);
#5062=VECTOR('',#17365,10.);
#5063=VECTOR('',#17366,10.);
#5064=VECTOR('',#17367,10.);
#5065=VECTOR('',#17370,10.);
#5066=VECTOR('',#17377,10.);
#5067=VECTOR('',#17378,10.);
#5068=VECTOR('',#17379,10.);
#5069=VECTOR('',#17382,10.);
#5070=VECTOR('',#17389,10.);
#5071=VECTOR('',#17390,10.);
#5072=VECTOR('',#17393,10.);
#5073=VECTOR('',#17394,10.);
#5074=VECTOR('',#17397,10.);
#5075=VECTOR('',#17400,10.);
#5076=VECTOR('',#17403,10.);
#5077=VECTOR('',#17408,10.);
#5078=VECTOR('',#17411,10.);
#5079=VECTOR('',#17414,10.);
#5080=VECTOR('',#17417,10.);
#5081=VECTOR('',#17420,10.);
#5082=VECTOR('',#17421,10.);
#5083=VECTOR('',#17426,10.);
#5084=VECTOR('',#17427,10.);
#5085=VECTOR('',#17430,10.);
#5086=VECTOR('',#17435,10.);
#5087=VECTOR('',#17436,10.);
#5088=VECTOR('',#17439,10.);
#5089=VECTOR('',#17444,10.);
#5090=VECTOR('',#17445,10.);
#5091=VECTOR('',#17448,10.);
#5092=VECTOR('',#17453,10.);
#5093=VECTOR('',#17456,10.);
#5094=VECTOR('',#17457,10.);
#5095=VECTOR('',#17458,10.);
#5096=VECTOR('',#17459,10.);
#5097=VECTOR('',#17460,10.);
#5098=VECTOR('',#17463,10.);
#5099=VECTOR('',#17468,10.);
#5100=VECTOR('',#17469,10.);
#5101=VECTOR('',#17470,10.);
#5102=VECTOR('',#17471,10.);
#5103=VECTOR('',#17474,10.);
#5104=VECTOR('',#17477,10.);
#5105=VECTOR('',#17478,10.);
#5106=VECTOR('',#17481,10.);
#5107=VECTOR('',#17484,10.);
#5108=VECTOR('',#17487,10.);
#5109=VECTOR('',#17490,10.);
#5110=VECTOR('',#17493,10.);
#5111=VECTOR('',#17494,10.);
#5112=VECTOR('',#17495,10.);
#5113=VECTOR('',#17496,10.);
#5114=VECTOR('',#17499,10.);
#5115=VECTOR('',#17502,10.);
#5116=VECTOR('',#17505,10.);
#5117=VECTOR('',#17508,10.);
#5118=VECTOR('',#17509,10.);
#5119=VECTOR('',#17512,10.);
#5120=VECTOR('',#17515,10.);
#5121=VECTOR('',#17518,10.);
#5122=VECTOR('',#17521,10.);
#5123=VECTOR('',#17524,10.);
#5124=VECTOR('',#17525,10.);
#5125=VECTOR('',#17528,10.);
#5126=VECTOR('',#17533,10.);
#5127=VECTOR('',#17534,10.);
#5128=VECTOR('',#17537,10.);
#5129=VECTOR('',#17544,10.);
#5130=VECTOR('',#17545,10.);
#5131=VECTOR('',#17546,10.);
#5132=VECTOR('',#17549,10.);
#5133=VECTOR('',#17556,10.);
#5134=VECTOR('',#17557,10.);
#5135=VECTOR('',#17562,10.);
#5136=VECTOR('',#17565,10.);
#5137=VECTOR('',#17566,10.);
#5138=VECTOR('',#17569,10.);
#5139=VECTOR('',#17570,10.);
#5140=VECTOR('',#17571,10.);
#5141=VECTOR('',#17574,10.);
#5142=VECTOR('',#17575,10.);
#5143=VECTOR('',#17578,10.);
#5144=VECTOR('',#17579,10.);
#5145=VECTOR('',#17580,10.);
#5146=VECTOR('',#17583,10.);
#5147=VECTOR('',#17588,10.);
#5148=VECTOR('',#17591,10.);
#5149=VECTOR('',#17594,10.);
#5150=VECTOR('',#17599,10.);
#5151=VECTOR('',#17600,10.);
#5152=VECTOR('',#17603,10.);
#6298=VERTEX_POINT('',#26846);
#6299=VERTEX_POINT('',#26847);
#6300=VERTEX_POINT('',#26849);
#6301=VERTEX_POINT('',#26851);
#6302=VERTEX_POINT('',#26855);
#6303=VERTEX_POINT('',#26856);
#6304=VERTEX_POINT('',#26861);
#6305=VERTEX_POINT('',#26862);
#6306=VERTEX_POINT('',#26867);
#6307=VERTEX_POINT('',#26868);
#6308=VERTEX_POINT('',#26873);
#6309=VERTEX_POINT('',#26874);
#6310=VERTEX_POINT('',#26879);
#6311=VERTEX_POINT('',#26880);
#6312=VERTEX_POINT('',#26885);
#6313=VERTEX_POINT('',#26886);
#6314=VERTEX_POINT('',#26894);
#6315=VERTEX_POINT('',#26896);
#6316=VERTEX_POINT('',#26900);
#6317=VERTEX_POINT('',#26904);
#6318=VERTEX_POINT('',#26908);
#6319=VERTEX_POINT('',#26912);
#6320=VERTEX_POINT('',#26913);
#6321=VERTEX_POINT('',#26915);
#6322=VERTEX_POINT('',#26917);
#6323=VERTEX_POINT('',#26919);
#6324=VERTEX_POINT('',#26921);
#6325=VERTEX_POINT('',#26923);
#6326=VERTEX_POINT('',#26925);
#6327=VERTEX_POINT('',#26929);
#6328=VERTEX_POINT('',#26930);
#6329=VERTEX_POINT('',#26932);
#6330=VERTEX_POINT('',#26934);
#6331=VERTEX_POINT('',#26938);
#6332=VERTEX_POINT('',#26939);
#6333=VERTEX_POINT('',#26944);
#6334=VERTEX_POINT('',#26945);
#6335=VERTEX_POINT('',#26950);
#6336=VERTEX_POINT('',#26951);
#6337=VERTEX_POINT('',#26956);
#6338=VERTEX_POINT('',#26957);
#6339=VERTEX_POINT('',#26962);
#6340=VERTEX_POINT('',#26963);
#6341=VERTEX_POINT('',#26968);
#6342=VERTEX_POINT('',#26969);
#6343=VERTEX_POINT('',#26986);
#6344=VERTEX_POINT('',#26987);
#6345=VERTEX_POINT('',#26989);
#6346=VERTEX_POINT('',#26991);
#6347=VERTEX_POINT('',#26993);
#6348=VERTEX_POINT('',#26995);
#6349=VERTEX_POINT('',#26997);
#6350=VERTEX_POINT('',#26999);
#6351=VERTEX_POINT('',#27003);
#6352=VERTEX_POINT('',#27005);
#6353=VERTEX_POINT('',#27009);
#6354=VERTEX_POINT('',#27013);
#6355=VERTEX_POINT('',#27017);
#6356=VERTEX_POINT('',#27021);
#6357=VERTEX_POINT('',#27025);
#6358=VERTEX_POINT('',#27029);
#6359=VERTEX_POINT('',#27035);
#6360=VERTEX_POINT('',#27037);
#6361=VERTEX_POINT('',#27039);
#6362=VERTEX_POINT('',#27041);
#6363=VERTEX_POINT('',#27045);
#6364=VERTEX_POINT('',#27047);
#6365=VERTEX_POINT('',#27115);
#6366=VERTEX_POINT('',#27121);
#6367=VERTEX_POINT('',#27126);
#6368=VERTEX_POINT('',#27128);
#6369=VERTEX_POINT('',#27133);
#6370=VERTEX_POINT('',#27209);
#6371=VERTEX_POINT('',#27211);
#6372=VERTEX_POINT('',#27213);
#6373=VERTEX_POINT('',#27217);
#6374=VERTEX_POINT('',#27219);
#6375=VERTEX_POINT('',#27287);
#6376=VERTEX_POINT('',#27294);
#6377=VERTEX_POINT('',#27299);
#6378=VERTEX_POINT('',#27301);
#6379=VERTEX_POINT('',#27306);
#6380=VERTEX_POINT('',#27419);
#6381=VERTEX_POINT('',#27517);
#6382=VERTEX_POINT('',#27629);
#6383=VERTEX_POINT('',#27630);
#6384=VERTEX_POINT('',#27698);
#6385=VERTEX_POINT('',#27703);
#6386=VERTEX_POINT('',#27822);
#6387=VERTEX_POINT('',#27828);
#6388=VERTEX_POINT('',#27836);
#6389=VERTEX_POINT('',#27837);
#6390=VERTEX_POINT('',#27839);
#6391=VERTEX_POINT('',#27841);
#6392=VERTEX_POINT('',#27900);
#6393=VERTEX_POINT('',#27909);
#6394=VERTEX_POINT('',#27944);
#6395=VERTEX_POINT('',#28042);
#6396=VERTEX_POINT('',#28093);
#6397=VERTEX_POINT('',#28094);
#6398=VERTEX_POINT('',#28192);
#6399=VERTEX_POINT('',#28197);
#6400=VERTEX_POINT('',#28306);
#6401=VERTEX_POINT('',#28307);
#6402=VERTEX_POINT('',#28375);
#6403=VERTEX_POINT('',#28380);
#6404=VERTEX_POINT('',#28511);
#6405=VERTEX_POINT('',#28520);
#6406=VERTEX_POINT('',#28531);
#6407=VERTEX_POINT('',#28532);
#6408=VERTEX_POINT('',#28534);
#6409=VERTEX_POINT('',#28536);
#6410=VERTEX_POINT('',#28583);
#6411=VERTEX_POINT('',#28589);
#6412=VERTEX_POINT('',#28628);
#6413=VERTEX_POINT('',#28630);
#6414=VERTEX_POINT('',#28634);
#6415=VERTEX_POINT('',#28638);
#6416=VERTEX_POINT('',#28642);
#6417=VERTEX_POINT('',#28646);
#6418=VERTEX_POINT('',#28647);
#6419=VERTEX_POINT('',#28652);
#6420=VERTEX_POINT('',#28653);
#6421=VERTEX_POINT('',#28658);
#6422=VERTEX_POINT('',#28659);
#6423=VERTEX_POINT('',#28667);
#6424=VERTEX_POINT('',#28672);
#6425=VERTEX_POINT('',#28674);
#6426=VERTEX_POINT('',#28679);
#6427=VERTEX_POINT('',#28681);
#6428=VERTEX_POINT('',#28686);
#6429=VERTEX_POINT('',#28688);
#6430=VERTEX_POINT('',#28734);
#6431=VERTEX_POINT('',#28971);
#6432=VERTEX_POINT('',#29114);
#6433=VERTEX_POINT('',#29115);
#8002=EDGE_CURVE('',#6298,#6299,#3718,.T.);
#8003=EDGE_CURVE('',#6299,#6300,#3719,.T.);
#8004=EDGE_CURVE('',#6300,#6301,#3720,.T.);
#8005=EDGE_CURVE('',#6301,#6298,#3721,.T.);
#8006=EDGE_CURVE('',#6302,#6303,#3722,.T.);
#8007=EDGE_CURVE('',#6303,#6299,#1021,.T.);
#8008=EDGE_CURVE('',#6298,#6302,#1022,.T.);
#8009=EDGE_CURVE('',#6304,#6305,#3723,.T.);
#8010=EDGE_CURVE('',#6305,#6303,#3724,.T.);
#8011=EDGE_CURVE('',#6302,#6304,#3725,.T.);
#8012=EDGE_CURVE('',#6306,#6307,#3726,.T.);
#8013=EDGE_CURVE('',#6307,#6305,#1023,.T.);
#8014=EDGE_CURVE('',#6304,#6306,#1024,.T.);
#8015=EDGE_CURVE('',#6308,#6309,#3727,.T.);
#8016=EDGE_CURVE('',#6309,#6307,#3728,.T.);
#8017=EDGE_CURVE('',#6306,#6308,#3729,.T.);
#8018=EDGE_CURVE('',#6310,#6311,#3730,.T.);
#8019=EDGE_CURVE('',#6311,#6309,#1025,.T.);
#8020=EDGE_CURVE('',#6308,#6310,#1026,.T.);
#8021=EDGE_CURVE('',#6312,#6313,#3731,.T.);
#8022=EDGE_CURVE('',#6313,#6311,#3732,.T.);
#8023=EDGE_CURVE('',#6310,#6312,#3733,.T.);
#8024=EDGE_CURVE('',#6300,#6313,#1027,.T.);
#8025=EDGE_CURVE('',#6312,#6301,#1028,.T.);
#8026=EDGE_CURVE('',#6304,#6314,#3734,.T.);
#8027=EDGE_CURVE('',#6315,#6314,#1029,.T.);
#8028=EDGE_CURVE('',#6306,#6315,#3735,.T.);
#8029=EDGE_CURVE('',#6302,#6316,#3736,.T.);
#8030=EDGE_CURVE('',#6314,#6316,#3737,.T.);
#8031=EDGE_CURVE('',#6298,#6317,#3738,.T.);
#8032=EDGE_CURVE('',#6316,#6317,#1030,.T.);
#8033=EDGE_CURVE('',#6301,#6318,#3739,.T.);
#8034=EDGE_CURVE('',#6317,#6318,#3740,.T.);
#8035=EDGE_CURVE('',#6319,#6320,#3741,.T.);
#8036=EDGE_CURVE('',#6321,#6319,#1031,.T.);
#8037=EDGE_CURVE('',#6322,#6321,#3742,.T.);
#8038=EDGE_CURVE('',#6323,#6322,#1032,.T.);
#8039=EDGE_CURVE('',#6324,#6323,#3743,.T.);
#8040=EDGE_CURVE('',#6325,#6324,#1033,.T.);
#8041=EDGE_CURVE('',#6326,#6325,#3744,.T.);
#8042=EDGE_CURVE('',#6320,#6326,#1034,.T.);
#8043=EDGE_CURVE('',#6327,#6328,#3745,.T.);
#8044=EDGE_CURVE('',#6328,#6329,#1035,.T.);
#8045=EDGE_CURVE('',#6329,#6330,#3746,.T.);
#8046=EDGE_CURVE('',#6330,#6327,#1036,.T.);
#8047=EDGE_CURVE('',#6331,#6332,#3747,.T.);
#8048=EDGE_CURVE('',#6332,#6328,#3748,.T.);
#8049=EDGE_CURVE('',#6327,#6331,#3749,.T.);
#8050=EDGE_CURVE('',#6333,#6334,#3750,.T.);
#8051=EDGE_CURVE('',#6334,#6332,#1037,.T.);
#8052=EDGE_CURVE('',#6331,#6333,#1038,.T.);
#8053=EDGE_CURVE('',#6335,#6336,#3751,.T.);
#8054=EDGE_CURVE('',#6336,#6334,#3752,.T.);
#8055=EDGE_CURVE('',#6333,#6335,#3753,.T.);
#8056=EDGE_CURVE('',#6337,#6338,#3754,.T.);
#8057=EDGE_CURVE('',#6338,#6336,#1039,.T.);
#8058=EDGE_CURVE('',#6335,#6337,#1040,.T.);
#8059=EDGE_CURVE('',#6339,#6340,#3755,.T.);
#8060=EDGE_CURVE('',#6340,#6338,#3756,.T.);
#8061=EDGE_CURVE('',#6337,#6339,#3757,.T.);
#8062=EDGE_CURVE('',#6341,#6342,#3758,.T.);
#8063=EDGE_CURVE('',#6342,#6340,#1041,.T.);
#8064=EDGE_CURVE('',#6339,#6341,#1042,.T.);
#8065=EDGE_CURVE('',#6329,#6342,#3759,.T.);
#8066=EDGE_CURVE('',#6341,#6330,#3760,.T.);
#8067=EDGE_CURVE('',#6333,#6326,#3761,.T.);
#8068=EDGE_CURVE('',#6335,#6325,#3762,.T.);
#8069=EDGE_CURVE('',#6331,#6320,#3763,.T.);
#8070=EDGE_CURVE('',#6327,#6319,#3764,.T.);
#8071=EDGE_CURVE('',#6330,#6321,#3765,.T.);
#8072=EDGE_CURVE('',#6343,#6344,#1043,.T.);
#8073=EDGE_CURVE('',#6345,#6343,#3766,.T.);
#8074=EDGE_CURVE('',#6346,#6345,#1044,.T.);
#8075=EDGE_CURVE('',#6347,#6346,#3767,.T.);
#8076=EDGE_CURVE('',#6348,#6347,#1045,.T.);
#8077=EDGE_CURVE('',#6349,#6348,#3768,.T.);
#8078=EDGE_CURVE('',#6350,#6349,#1046,.T.);
#8079=EDGE_CURVE('',#6344,#6350,#3769,.T.);
#8080=EDGE_CURVE('',#6351,#6343,#3770,.T.);
#8081=EDGE_CURVE('',#6344,#6352,#3771,.T.);
#8082=EDGE_CURVE('',#6352,#6351,#1047,.T.);
#8083=EDGE_CURVE('',#6351,#6353,#3772,.T.);
#8084=EDGE_CURVE('',#6353,#6345,#3773,.T.);
#8085=EDGE_CURVE('',#6354,#6346,#3774,.T.);
#8086=EDGE_CURVE('',#6353,#6354,#1048,.T.);
#8087=EDGE_CURVE('',#6354,#6355,#3775,.T.);
#8088=EDGE_CURVE('',#6355,#6347,#3776,.T.);
#8089=EDGE_CURVE('',#6356,#6348,#3777,.T.);
#8090=EDGE_CURVE('',#6355,#6356,#1049,.T.);
#8091=EDGE_CURVE('',#6356,#6357,#3778,.T.);
#8092=EDGE_CURVE('',#6357,#6349,#3779,.T.);
#8093=EDGE_CURVE('',#6358,#6350,#3780,.T.);
#8094=EDGE_CURVE('',#6357,#6358,#1050,.T.);
#8095=EDGE_CURVE('',#6358,#6352,#3781,.T.);
#8096=EDGE_CURVE('',#6354,#6359,#3782,.T.);
#8097=EDGE_CURVE('',#6360,#6359,#3783,.T.);
#8098=EDGE_CURVE('',#6361,#6360,#3784,.T.);
#8099=EDGE_CURVE('',#6362,#6361,#3785,.T.);
#8100=EDGE_CURVE('',#6355,#6362,#3786,.T.);
#8101=EDGE_CURVE('',#6353,#6363,#3787,.T.);
#8102=EDGE_CURVE('',#6364,#6363,#296,.T.);
#8103=EDGE_CURVE('',#6365,#6364,#297,.T.);
#8104=EDGE_CURVE('',#6366,#6365,#298,.T.);
#8105=EDGE_CURVE('',#6367,#6366,#1051,.T.);
#8106=EDGE_CURVE('',#6368,#6367,#299,.T.);
#8107=EDGE_CURVE('',#6369,#6368,#300,.T.);
#8108=EDGE_CURVE('',#6359,#6369,#301,.T.);
#8109=EDGE_CURVE('',#6351,#6370,#3788,.T.);
#8110=EDGE_CURVE('',#6371,#6370,#3789,.T.);
#8111=EDGE_CURVE('',#6372,#6371,#3790,.T.);
#8112=EDGE_CURVE('',#6363,#6372,#3791,.T.);
#8113=EDGE_CURVE('',#6352,#6373,#3792,.T.);
#8114=EDGE_CURVE('',#6374,#6373,#302,.T.);
#8115=EDGE_CURVE('',#6375,#6374,#303,.T.);
#8116=EDGE_CURVE('',#6376,#6375,#304,.T.);
#8117=EDGE_CURVE('',#6377,#6376,#1052,.T.);
#8118=EDGE_CURVE('',#6378,#6377,#305,.T.);
#8119=EDGE_CURVE('',#6379,#6378,#306,.T.);
#8120=EDGE_CURVE('',#6370,#6379,#307,.T.);
#8121=EDGE_CURVE('',#6361,#6380,#308,.T.);
#8122=EDGE_CURVE('',#6381,#6380,#309,.T.);
#8123=EDGE_CURVE('',#6381,#6362,#310,.T.);
#8124=EDGE_CURVE('',#6382,#6383,#311,.T.);
#8125=EDGE_CURVE('',#6384,#6383,#312,.T.);
#8126=EDGE_CURVE('',#6384,#6385,#313,.T.);
#8127=EDGE_CURVE('',#6385,#6382,#3793,.T.);
#8128=EDGE_CURVE('',#6383,#6386,#314,.T.);
#8129=EDGE_CURVE('',#6386,#6387,#3794,.T.);
#8130=EDGE_CURVE('',#6387,#6384,#315,.T.);
#8131=EDGE_CURVE('',#6388,#6389,#3795,.T.);
#8132=EDGE_CURVE('',#6389,#6390,#1053,.T.);
#8133=EDGE_CURVE('',#6390,#6391,#3796,.T.);
#8134=EDGE_CURVE('',#6391,#6388,#1054,.T.);
#8135=EDGE_CURVE('',#6390,#6387,#316,.T.);
#8136=EDGE_CURVE('',#6386,#6391,#317,.T.);
#8137=EDGE_CURVE('',#6380,#6392,#318,.T.);
#8138=EDGE_CURVE('',#6392,#6393,#3797,.T.);
#8139=EDGE_CURVE('',#6393,#6381,#319,.T.);
#8140=EDGE_CURVE('',#6392,#6389,#320,.T.);
#8141=EDGE_CURVE('',#6388,#6393,#321,.T.);
#8142=EDGE_CURVE('',#6394,#6360,#322,.T.);
#8143=EDGE_CURVE('',#6395,#6394,#323,.T.);
#8144=EDGE_CURVE('',#6395,#6392,#3798,.T.);
#8145=EDGE_CURVE('',#6356,#6382,#3799,.T.);
#8146=EDGE_CURVE('',#6396,#6397,#324,.T.);
#8147=EDGE_CURVE('',#6398,#6397,#325,.T.);
#8148=EDGE_CURVE('',#6398,#6399,#326,.T.);
#8149=EDGE_CURVE('',#6399,#6396,#3800,.T.);
#8150=EDGE_CURVE('',#6400,#6401,#327,.T.);
#8151=EDGE_CURVE('',#6402,#6401,#328,.T.);
#8152=EDGE_CURVE('',#6402,#6403,#329,.T.);
#8153=EDGE_CURVE('',#6403,#6400,#3801,.T.);
#8154=EDGE_CURVE('',#6401,#6404,#330,.T.);
#8155=EDGE_CURVE('',#6404,#6405,#3802,.T.);
#8156=EDGE_CURVE('',#6405,#6402,#331,.T.);
#8157=EDGE_CURVE('',#6406,#6407,#3803,.T.);
#8158=EDGE_CURVE('',#6407,#6408,#1055,.T.);
#8159=EDGE_CURVE('',#6408,#6409,#3804,.T.);
#8160=EDGE_CURVE('',#6409,#6406,#1056,.T.);
#8161=EDGE_CURVE('',#6408,#6405,#332,.T.);
#8162=EDGE_CURVE('',#6404,#6409,#333,.T.);
#8163=EDGE_CURVE('',#6397,#6410,#334,.T.);
#8164=EDGE_CURVE('',#6410,#6411,#3805,.T.);
#8165=EDGE_CURVE('',#6411,#6398,#335,.T.);
#8166=EDGE_CURVE('',#6410,#6407,#336,.T.);
#8167=EDGE_CURVE('',#6406,#6411,#337,.T.);
#8168=EDGE_CURVE('',#6387,#6410,#3806,.T.);
#8169=EDGE_CURVE('',#6396,#6385,#3807,.T.);
#8170=EDGE_CURVE('',#6357,#6399,#3808,.T.);
#8171=EDGE_CURVE('',#6358,#6400,#3809,.T.);
#8172=EDGE_CURVE('',#6314,#6412,#3810,.T.);
#8173=EDGE_CURVE('',#6412,#6413,#1057,.T.);
#8174=EDGE_CURVE('',#6413,#6315,#3811,.T.);
#8175=EDGE_CURVE('',#6316,#6414,#3812,.T.);
#8176=EDGE_CURVE('',#6414,#6412,#3813,.T.);
#8177=EDGE_CURVE('',#6317,#6415,#3814,.T.);
#8178=EDGE_CURVE('',#6415,#6414,#1058,.T.);
#8179=EDGE_CURVE('',#6318,#6416,#3815,.T.);
#8180=EDGE_CURVE('',#6416,#6415,#3816,.T.);
#8181=EDGE_CURVE('',#6417,#6418,#3817,.T.);
#8182=EDGE_CURVE('',#6418,#6416,#1059,.T.);
#8183=EDGE_CURVE('',#6318,#6417,#1060,.T.);
#8184=EDGE_CURVE('',#6419,#6420,#3818,.T.);
#8185=EDGE_CURVE('',#6420,#6418,#3819,.T.);
#8186=EDGE_CURVE('',#6417,#6419,#3820,.T.);
#8187=EDGE_CURVE('',#6421,#6422,#3821,.T.);
#8188=EDGE_CURVE('',#6422,#6420,#1061,.T.);
#8189=EDGE_CURVE('',#6419,#6421,#1062,.T.);
#8190=EDGE_CURVE('',#6413,#6422,#3822,.T.);
#8191=EDGE_CURVE('',#6421,#6315,#3823,.T.);
#8192=EDGE_CURVE('',#6423,#6395,#338,.T.);
#8193=EDGE_CURVE('',#6424,#6423,#1063,.T.);
#8194=EDGE_CURVE('',#6425,#6424,#339,.T.);
#8195=EDGE_CURVE('',#6426,#6425,#3824,.T.);
#8196=EDGE_CURVE('',#6427,#6426,#340,.T.);
#8197=EDGE_CURVE('',#6428,#6427,#1064,.T.);
#8198=EDGE_CURVE('',#6429,#6428,#341,.T.);
#8199=EDGE_CURVE('',#6405,#6429,#3825,.T.);
#8200=EDGE_CURVE('',#6372,#6430,#342,.T.);
#8201=EDGE_CURVE('',#6364,#6430,#343,.T.);
#8202=EDGE_CURVE('',#6394,#6369,#344,.T.);
#8203=EDGE_CURVE('',#6368,#6395,#3826,.T.);
#8204=EDGE_CURVE('',#6366,#6424,#3827,.T.);
#8205=EDGE_CURVE('',#6423,#6367,#3828,.T.);
#8206=EDGE_CURVE('',#6430,#6425,#345,.T.);
#8207=EDGE_CURVE('',#6425,#6365,#3829,.T.);
#8208=EDGE_CURVE('',#6431,#6371,#346,.T.);
#8209=EDGE_CURVE('',#6426,#6431,#347,.T.);
#8210=EDGE_CURVE('',#6432,#6433,#348,.T.);
#8211=EDGE_CURVE('',#6374,#6433,#349,.T.);
#8212=EDGE_CURVE('',#6373,#6432,#3830,.T.);
#8213=EDGE_CURVE('',#6431,#6379,#350,.T.);
#8214=EDGE_CURVE('',#6378,#6426,#3831,.T.);
#8215=EDGE_CURVE('',#6376,#6428,#3832,.T.);
#8216=EDGE_CURVE('',#6427,#6377,#3833,.T.);
#8217=EDGE_CURVE('',#6433,#6429,#351,.T.);
#8218=EDGE_CURVE('',#6429,#6375,#3834,.T.);
#8219=EDGE_CURVE('',#6432,#6403,#3835,.T.);
#8220=EDGE_CURVE('',#6308,#6421,#3836,.T.);
#8221=EDGE_CURVE('',#6310,#6419,#3837,.T.);
#8222=EDGE_CURVE('',#6312,#6417,#3838,.T.);
#8223=EDGE_CURVE('',#6337,#6324,#3839,.T.);
#8224=EDGE_CURVE('',#6339,#6323,#3840,.T.);
#8225=EDGE_CURVE('',#6341,#6322,#3841,.T.);
#11251=ORIENTED_EDGE('',*,*,#8002,.T.);
#11252=ORIENTED_EDGE('',*,*,#8003,.T.);
#11253=ORIENTED_EDGE('',*,*,#8004,.T.);
#11254=ORIENTED_EDGE('',*,*,#8005,.T.);
#11255=ORIENTED_EDGE('',*,*,#8006,.T.);
#11256=ORIENTED_EDGE('',*,*,#8007,.T.);
#11257=ORIENTED_EDGE('',*,*,#8002,.F.);
#11258=ORIENTED_EDGE('',*,*,#8008,.T.);
#11259=ORIENTED_EDGE('',*,*,#8009,.T.);
#11260=ORIENTED_EDGE('',*,*,#8010,.T.);
#11261=ORIENTED_EDGE('',*,*,#8006,.F.);
#11262=ORIENTED_EDGE('',*,*,#8011,.T.);
#11263=ORIENTED_EDGE('',*,*,#8012,.T.);
#11264=ORIENTED_EDGE('',*,*,#8013,.T.);
#11265=ORIENTED_EDGE('',*,*,#8009,.F.);
#11266=ORIENTED_EDGE('',*,*,#8014,.T.);
#11267=ORIENTED_EDGE('',*,*,#8015,.T.);
#11268=ORIENTED_EDGE('',*,*,#8016,.T.);
#11269=ORIENTED_EDGE('',*,*,#8012,.F.);
#11270=ORIENTED_EDGE('',*,*,#8017,.T.);
#11271=ORIENTED_EDGE('',*,*,#8018,.T.);
#11272=ORIENTED_EDGE('',*,*,#8019,.T.);
#11273=ORIENTED_EDGE('',*,*,#8015,.F.);
#11274=ORIENTED_EDGE('',*,*,#8020,.T.);
#11275=ORIENTED_EDGE('',*,*,#8021,.T.);
#11276=ORIENTED_EDGE('',*,*,#8022,.T.);
#11277=ORIENTED_EDGE('',*,*,#8018,.F.);
#11278=ORIENTED_EDGE('',*,*,#8023,.T.);
#11279=ORIENTED_EDGE('',*,*,#8004,.F.);
#11280=ORIENTED_EDGE('',*,*,#8024,.T.);
#11281=ORIENTED_EDGE('',*,*,#8021,.F.);
#11282=ORIENTED_EDGE('',*,*,#8025,.T.);
#11283=ORIENTED_EDGE('',*,*,#8014,.F.);
#11284=ORIENTED_EDGE('',*,*,#8026,.T.);
#11285=ORIENTED_EDGE('',*,*,#8027,.F.);
#11286=ORIENTED_EDGE('',*,*,#8028,.F.);
#11287=ORIENTED_EDGE('',*,*,#8011,.F.);
#11288=ORIENTED_EDGE('',*,*,#8029,.T.);
#11289=ORIENTED_EDGE('',*,*,#8030,.F.);
#11290=ORIENTED_EDGE('',*,*,#8026,.F.);
#11291=ORIENTED_EDGE('',*,*,#8008,.F.);
#11292=ORIENTED_EDGE('',*,*,#8031,.T.);
#11293=ORIENTED_EDGE('',*,*,#8032,.F.);
#11294=ORIENTED_EDGE('',*,*,#8029,.F.);
#11295=ORIENTED_EDGE('',*,*,#8005,.F.);
#11296=ORIENTED_EDGE('',*,*,#8033,.T.);
#11297=ORIENTED_EDGE('',*,*,#8034,.F.);
#11298=ORIENTED_EDGE('',*,*,#8031,.F.);
#11299=ORIENTED_EDGE('',*,*,#8035,.F.);
#11300=ORIENTED_EDGE('',*,*,#8036,.F.);
#11301=ORIENTED_EDGE('',*,*,#8037,.F.);
#11302=ORIENTED_EDGE('',*,*,#8038,.F.);
#11303=ORIENTED_EDGE('',*,*,#8039,.F.);
#11304=ORIENTED_EDGE('',*,*,#8040,.F.);
#11305=ORIENTED_EDGE('',*,*,#8041,.F.);
#11306=ORIENTED_EDGE('',*,*,#8042,.F.);
#11307=ORIENTED_EDGE('',*,*,#8003,.F.);
#11308=ORIENTED_EDGE('',*,*,#8007,.F.);
#11309=ORIENTED_EDGE('',*,*,#8010,.F.);
#11310=ORIENTED_EDGE('',*,*,#8013,.F.);
#11311=ORIENTED_EDGE('',*,*,#8016,.F.);
#11312=ORIENTED_EDGE('',*,*,#8019,.F.);
#11313=ORIENTED_EDGE('',*,*,#8022,.F.);
#11314=ORIENTED_EDGE('',*,*,#8024,.F.);
#11315=ORIENTED_EDGE('',*,*,#8043,.T.);
#11316=ORIENTED_EDGE('',*,*,#8044,.T.);
#11317=ORIENTED_EDGE('',*,*,#8045,.T.);
#11318=ORIENTED_EDGE('',*,*,#8046,.T.);
#11319=ORIENTED_EDGE('',*,*,#8047,.T.);
#11320=ORIENTED_EDGE('',*,*,#8048,.T.);
#11321=ORIENTED_EDGE('',*,*,#8043,.F.);
#11322=ORIENTED_EDGE('',*,*,#8049,.T.);
#11323=ORIENTED_EDGE('',*,*,#8050,.T.);
#11324=ORIENTED_EDGE('',*,*,#8051,.T.);
#11325=ORIENTED_EDGE('',*,*,#8047,.F.);
#11326=ORIENTED_EDGE('',*,*,#8052,.T.);
#11327=ORIENTED_EDGE('',*,*,#8053,.T.);
#11328=ORIENTED_EDGE('',*,*,#8054,.T.);
#11329=ORIENTED_EDGE('',*,*,#8050,.F.);
#11330=ORIENTED_EDGE('',*,*,#8055,.T.);
#11331=ORIENTED_EDGE('',*,*,#8056,.T.);
#11332=ORIENTED_EDGE('',*,*,#8057,.T.);
#11333=ORIENTED_EDGE('',*,*,#8053,.F.);
#11334=ORIENTED_EDGE('',*,*,#8058,.T.);
#11335=ORIENTED_EDGE('',*,*,#8059,.T.);
#11336=ORIENTED_EDGE('',*,*,#8060,.T.);
#11337=ORIENTED_EDGE('',*,*,#8056,.F.);
#11338=ORIENTED_EDGE('',*,*,#8061,.T.);
#11339=ORIENTED_EDGE('',*,*,#8062,.T.);
#11340=ORIENTED_EDGE('',*,*,#8063,.T.);
#11341=ORIENTED_EDGE('',*,*,#8059,.F.);
#11342=ORIENTED_EDGE('',*,*,#8064,.T.);
#11343=ORIENTED_EDGE('',*,*,#8045,.F.);
#11344=ORIENTED_EDGE('',*,*,#8065,.T.);
#11345=ORIENTED_EDGE('',*,*,#8062,.F.);
#11346=ORIENTED_EDGE('',*,*,#8066,.T.);
#11347=ORIENTED_EDGE('',*,*,#8055,.F.);
#11348=ORIENTED_EDGE('',*,*,#8067,.T.);
#11349=ORIENTED_EDGE('',*,*,#8041,.T.);
#11350=ORIENTED_EDGE('',*,*,#8068,.F.);
#11351=ORIENTED_EDGE('',*,*,#8052,.F.);
#11352=ORIENTED_EDGE('',*,*,#8069,.T.);
#11353=ORIENTED_EDGE('',*,*,#8042,.T.);
#11354=ORIENTED_EDGE('',*,*,#8067,.F.);
#11355=ORIENTED_EDGE('',*,*,#8049,.F.);
#11356=ORIENTED_EDGE('',*,*,#8070,.T.);
#11357=ORIENTED_EDGE('',*,*,#8035,.T.);
#11358=ORIENTED_EDGE('',*,*,#8069,.F.);
#11359=ORIENTED_EDGE('',*,*,#8046,.F.);
#11360=ORIENTED_EDGE('',*,*,#8071,.T.);
#11361=ORIENTED_EDGE('',*,*,#8036,.T.);
#11362=ORIENTED_EDGE('',*,*,#8070,.F.);
#11363=ORIENTED_EDGE('',*,*,#8072,.F.);
#11364=ORIENTED_EDGE('',*,*,#8073,.F.);
#11365=ORIENTED_EDGE('',*,*,#8074,.F.);
#11366=ORIENTED_EDGE('',*,*,#8075,.F.);
#11367=ORIENTED_EDGE('',*,*,#8076,.F.);
#11368=ORIENTED_EDGE('',*,*,#8077,.F.);
#11369=ORIENTED_EDGE('',*,*,#8078,.F.);
#11370=ORIENTED_EDGE('',*,*,#8079,.F.);
#11371=ORIENTED_EDGE('',*,*,#8044,.F.);
#11372=ORIENTED_EDGE('',*,*,#8048,.F.);
#11373=ORIENTED_EDGE('',*,*,#8051,.F.);
#11374=ORIENTED_EDGE('',*,*,#8054,.F.);
#11375=ORIENTED_EDGE('',*,*,#8057,.F.);
#11376=ORIENTED_EDGE('',*,*,#8060,.F.);
#11377=ORIENTED_EDGE('',*,*,#8063,.F.);
#11378=ORIENTED_EDGE('',*,*,#8065,.F.);
#11379=ORIENTED_EDGE('',*,*,#8080,.T.);
#11380=ORIENTED_EDGE('',*,*,#8072,.T.);
#11381=ORIENTED_EDGE('',*,*,#8081,.T.);
#11382=ORIENTED_EDGE('',*,*,#8082,.T.);
#11383=ORIENTED_EDGE('',*,*,#8080,.F.);
#11384=ORIENTED_EDGE('',*,*,#8083,.T.);
#11385=ORIENTED_EDGE('',*,*,#8084,.T.);
#11386=ORIENTED_EDGE('',*,*,#8073,.T.);
#11387=ORIENTED_EDGE('',*,*,#8085,.T.);
#11388=ORIENTED_EDGE('',*,*,#8074,.T.);
#11389=ORIENTED_EDGE('',*,*,#8084,.F.);
#11390=ORIENTED_EDGE('',*,*,#8086,.T.);
#11391=ORIENTED_EDGE('',*,*,#8085,.F.);
#11392=ORIENTED_EDGE('',*,*,#8087,.T.);
#11393=ORIENTED_EDGE('',*,*,#8088,.T.);
#11394=ORIENTED_EDGE('',*,*,#8075,.T.);
#11395=ORIENTED_EDGE('',*,*,#8089,.T.);
#11396=ORIENTED_EDGE('',*,*,#8076,.T.);
#11397=ORIENTED_EDGE('',*,*,#8088,.F.);
#11398=ORIENTED_EDGE('',*,*,#8090,.T.);
#11399=ORIENTED_EDGE('',*,*,#8089,.F.);
#11400=ORIENTED_EDGE('',*,*,#8091,.T.);
#11401=ORIENTED_EDGE('',*,*,#8092,.T.);
#11402=ORIENTED_EDGE('',*,*,#8077,.T.);
#11403=ORIENTED_EDGE('',*,*,#8093,.T.);
#11404=ORIENTED_EDGE('',*,*,#8078,.T.);
#11405=ORIENTED_EDGE('',*,*,#8092,.F.);
#11406=ORIENTED_EDGE('',*,*,#8094,.T.);
#11407=ORIENTED_EDGE('',*,*,#8093,.F.);
#11408=ORIENTED_EDGE('',*,*,#8095,.T.);
#11409=ORIENTED_EDGE('',*,*,#8081,.F.);
#11410=ORIENTED_EDGE('',*,*,#8079,.T.);
#11411=ORIENTED_EDGE('',*,*,#8087,.F.);
#11412=ORIENTED_EDGE('',*,*,#8096,.T.);
#11413=ORIENTED_EDGE('',*,*,#8097,.F.);
#11414=ORIENTED_EDGE('',*,*,#8098,.F.);
#11415=ORIENTED_EDGE('',*,*,#8099,.F.);
#11416=ORIENTED_EDGE('',*,*,#8100,.F.);
#11417=ORIENTED_EDGE('',*,*,#8086,.F.);
#11418=ORIENTED_EDGE('',*,*,#8101,.T.);
#11419=ORIENTED_EDGE('',*,*,#8102,.F.);
#11420=ORIENTED_EDGE('',*,*,#8103,.F.);
#11421=ORIENTED_EDGE('',*,*,#8104,.F.);
#11422=ORIENTED_EDGE('',*,*,#8105,.F.);
#11423=ORIENTED_EDGE('',*,*,#8106,.F.);
#11424=ORIENTED_EDGE('',*,*,#8107,.F.);
#11425=ORIENTED_EDGE('',*,*,#8108,.F.);
#11426=ORIENTED_EDGE('',*,*,#8096,.F.);
#11427=ORIENTED_EDGE('',*,*,#8083,.F.);
#11428=ORIENTED_EDGE('',*,*,#8109,.T.);
#11429=ORIENTED_EDGE('',*,*,#8110,.F.);
#11430=ORIENTED_EDGE('',*,*,#8111,.F.);
#11431=ORIENTED_EDGE('',*,*,#8112,.F.);
#11432=ORIENTED_EDGE('',*,*,#8101,.F.);
#11433=ORIENTED_EDGE('',*,*,#8082,.F.);
#11434=ORIENTED_EDGE('',*,*,#8113,.T.);
#11435=ORIENTED_EDGE('',*,*,#8114,.F.);
#11436=ORIENTED_EDGE('',*,*,#8115,.F.);
#11437=ORIENTED_EDGE('',*,*,#8116,.F.);
#11438=ORIENTED_EDGE('',*,*,#8117,.F.);
#11439=ORIENTED_EDGE('',*,*,#8118,.F.);
#11440=ORIENTED_EDGE('',*,*,#8119,.F.);
#11441=ORIENTED_EDGE('',*,*,#8120,.F.);
#11442=ORIENTED_EDGE('',*,*,#8109,.F.);
#11443=ORIENTED_EDGE('',*,*,#8121,.T.);
#11444=ORIENTED_EDGE('',*,*,#8122,.F.);
#11445=ORIENTED_EDGE('',*,*,#8123,.T.);
#11446=ORIENTED_EDGE('',*,*,#8099,.T.);
#11447=ORIENTED_EDGE('',*,*,#8124,.T.);
#11448=ORIENTED_EDGE('',*,*,#8125,.F.);
#11449=ORIENTED_EDGE('',*,*,#8126,.T.);
#11450=ORIENTED_EDGE('',*,*,#8127,.T.);
#11451=ORIENTED_EDGE('',*,*,#8125,.T.);
#11452=ORIENTED_EDGE('',*,*,#8128,.T.);
#11453=ORIENTED_EDGE('',*,*,#8129,.T.);
#11454=ORIENTED_EDGE('',*,*,#8130,.T.);
#11455=ORIENTED_EDGE('',*,*,#8131,.T.);
#11456=ORIENTED_EDGE('',*,*,#8132,.T.);
#11457=ORIENTED_EDGE('',*,*,#8133,.T.);
#11458=ORIENTED_EDGE('',*,*,#8134,.T.);
#11459=ORIENTED_EDGE('',*,*,#8133,.F.);
#11460=ORIENTED_EDGE('',*,*,#8135,.T.);
#11461=ORIENTED_EDGE('',*,*,#8129,.F.);
#11462=ORIENTED_EDGE('',*,*,#8136,.T.);
#11463=ORIENTED_EDGE('',*,*,#8122,.T.);
#11464=ORIENTED_EDGE('',*,*,#8137,.T.);
#11465=ORIENTED_EDGE('',*,*,#8138,.T.);
#11466=ORIENTED_EDGE('',*,*,#8139,.T.);
#11467=ORIENTED_EDGE('',*,*,#8138,.F.);
#11468=ORIENTED_EDGE('',*,*,#8140,.T.);
#11469=ORIENTED_EDGE('',*,*,#8131,.F.);
#11470=ORIENTED_EDGE('',*,*,#8141,.T.);
#11471=ORIENTED_EDGE('',*,*,#8137,.F.);
#11472=ORIENTED_EDGE('',*,*,#8121,.F.);
#11473=ORIENTED_EDGE('',*,*,#8098,.T.);
#11474=ORIENTED_EDGE('',*,*,#8142,.F.);
#11475=ORIENTED_EDGE('',*,*,#8143,.F.);
#11476=ORIENTED_EDGE('',*,*,#8144,.T.);
#11477=ORIENTED_EDGE('',*,*,#8090,.F.);
#11478=ORIENTED_EDGE('',*,*,#8100,.T.);
#11479=ORIENTED_EDGE('',*,*,#8123,.F.);
#11480=ORIENTED_EDGE('',*,*,#8139,.F.);
#11481=ORIENTED_EDGE('',*,*,#8141,.F.);
#11482=ORIENTED_EDGE('',*,*,#8134,.F.);
#11483=ORIENTED_EDGE('',*,*,#8136,.F.);
#11484=ORIENTED_EDGE('',*,*,#8128,.F.);
#11485=ORIENTED_EDGE('',*,*,#8124,.F.);
#11486=ORIENTED_EDGE('',*,*,#8145,.F.);
#11487=ORIENTED_EDGE('',*,*,#8146,.T.);
#11488=ORIENTED_EDGE('',*,*,#8147,.F.);
#11489=ORIENTED_EDGE('',*,*,#8148,.T.);
#11490=ORIENTED_EDGE('',*,*,#8149,.T.);
#11491=ORIENTED_EDGE('',*,*,#8150,.T.);
#11492=ORIENTED_EDGE('',*,*,#8151,.F.);
#11493=ORIENTED_EDGE('',*,*,#8152,.T.);
#11494=ORIENTED_EDGE('',*,*,#8153,.T.);
#11495=ORIENTED_EDGE('',*,*,#8151,.T.);
#11496=ORIENTED_EDGE('',*,*,#8154,.T.);
#11497=ORIENTED_EDGE('',*,*,#8155,.T.);
#11498=ORIENTED_EDGE('',*,*,#8156,.T.);
#11499=ORIENTED_EDGE('',*,*,#8157,.T.);
#11500=ORIENTED_EDGE('',*,*,#8158,.T.);
#11501=ORIENTED_EDGE('',*,*,#8159,.T.);
#11502=ORIENTED_EDGE('',*,*,#8160,.T.);
#11503=ORIENTED_EDGE('',*,*,#8159,.F.);
#11504=ORIENTED_EDGE('',*,*,#8161,.T.);
#11505=ORIENTED_EDGE('',*,*,#8155,.F.);
#11506=ORIENTED_EDGE('',*,*,#8162,.T.);
#11507=ORIENTED_EDGE('',*,*,#8147,.T.);
#11508=ORIENTED_EDGE('',*,*,#8163,.T.);
#11509=ORIENTED_EDGE('',*,*,#8164,.T.);
#11510=ORIENTED_EDGE('',*,*,#8165,.T.);
#11511=ORIENTED_EDGE('',*,*,#8164,.F.);
#11512=ORIENTED_EDGE('',*,*,#8166,.T.);
#11513=ORIENTED_EDGE('',*,*,#8157,.F.);
#11514=ORIENTED_EDGE('',*,*,#8167,.T.);
#11515=ORIENTED_EDGE('',*,*,#8130,.F.);
#11516=ORIENTED_EDGE('',*,*,#8168,.T.);
#11517=ORIENTED_EDGE('',*,*,#8163,.F.);
#11518=ORIENTED_EDGE('',*,*,#8146,.F.);
#11519=ORIENTED_EDGE('',*,*,#8169,.T.);
#11520=ORIENTED_EDGE('',*,*,#8126,.F.);
#11521=ORIENTED_EDGE('',*,*,#8091,.F.);
#11522=ORIENTED_EDGE('',*,*,#8145,.T.);
#11523=ORIENTED_EDGE('',*,*,#8127,.F.);
#11524=ORIENTED_EDGE('',*,*,#8169,.F.);
#11525=ORIENTED_EDGE('',*,*,#8149,.F.);
#11526=ORIENTED_EDGE('',*,*,#8170,.F.);
#11527=ORIENTED_EDGE('',*,*,#8094,.F.);
#11528=ORIENTED_EDGE('',*,*,#8170,.T.);
#11529=ORIENTED_EDGE('',*,*,#8148,.F.);
#11530=ORIENTED_EDGE('',*,*,#8165,.F.);
#11531=ORIENTED_EDGE('',*,*,#8167,.F.);
#11532=ORIENTED_EDGE('',*,*,#8160,.F.);
#11533=ORIENTED_EDGE('',*,*,#8162,.F.);
#11534=ORIENTED_EDGE('',*,*,#8154,.F.);
#11535=ORIENTED_EDGE('',*,*,#8150,.F.);
#11536=ORIENTED_EDGE('',*,*,#8171,.F.);
#11537=ORIENTED_EDGE('',*,*,#8172,.T.);
#11538=ORIENTED_EDGE('',*,*,#8173,.T.);
#11539=ORIENTED_EDGE('',*,*,#8174,.T.);
#11540=ORIENTED_EDGE('',*,*,#8027,.T.);
#11541=ORIENTED_EDGE('',*,*,#8175,.T.);
#11542=ORIENTED_EDGE('',*,*,#8176,.T.);
#11543=ORIENTED_EDGE('',*,*,#8172,.F.);
#11544=ORIENTED_EDGE('',*,*,#8030,.T.);
#11545=ORIENTED_EDGE('',*,*,#8177,.T.);
#11546=ORIENTED_EDGE('',*,*,#8178,.T.);
#11547=ORIENTED_EDGE('',*,*,#8175,.F.);
#11548=ORIENTED_EDGE('',*,*,#8032,.T.);
#11549=ORIENTED_EDGE('',*,*,#8179,.T.);
#11550=ORIENTED_EDGE('',*,*,#8180,.T.);
#11551=ORIENTED_EDGE('',*,*,#8177,.F.);
#11552=ORIENTED_EDGE('',*,*,#8034,.T.);
#11553=ORIENTED_EDGE('',*,*,#8181,.T.);
#11554=ORIENTED_EDGE('',*,*,#8182,.T.);
#11555=ORIENTED_EDGE('',*,*,#8179,.F.);
#11556=ORIENTED_EDGE('',*,*,#8183,.T.);
#11557=ORIENTED_EDGE('',*,*,#8184,.T.);
#11558=ORIENTED_EDGE('',*,*,#8185,.T.);
#11559=ORIENTED_EDGE('',*,*,#8181,.F.);
#11560=ORIENTED_EDGE('',*,*,#8186,.T.);
#11561=ORIENTED_EDGE('',*,*,#8187,.T.);
#11562=ORIENTED_EDGE('',*,*,#8188,.T.);
#11563=ORIENTED_EDGE('',*,*,#8184,.F.);
#11564=ORIENTED_EDGE('',*,*,#8189,.T.);
#11565=ORIENTED_EDGE('',*,*,#8174,.F.);
#11566=ORIENTED_EDGE('',*,*,#8190,.T.);
#11567=ORIENTED_EDGE('',*,*,#8187,.F.);
#11568=ORIENTED_EDGE('',*,*,#8191,.T.);
#11569=ORIENTED_EDGE('',*,*,#8140,.F.);
#11570=ORIENTED_EDGE('',*,*,#8144,.F.);
#11571=ORIENTED_EDGE('',*,*,#8192,.F.);
#11572=ORIENTED_EDGE('',*,*,#8193,.F.);
#11573=ORIENTED_EDGE('',*,*,#8194,.F.);
#11574=ORIENTED_EDGE('',*,*,#8195,.F.);
#11575=ORIENTED_EDGE('',*,*,#8196,.F.);
#11576=ORIENTED_EDGE('',*,*,#8197,.F.);
#11577=ORIENTED_EDGE('',*,*,#8198,.F.);
#11578=ORIENTED_EDGE('',*,*,#8199,.F.);
#11579=ORIENTED_EDGE('',*,*,#8161,.F.);
#11580=ORIENTED_EDGE('',*,*,#8158,.F.);
#11581=ORIENTED_EDGE('',*,*,#8166,.F.);
#11582=ORIENTED_EDGE('',*,*,#8168,.F.);
#11583=ORIENTED_EDGE('',*,*,#8135,.F.);
#11584=ORIENTED_EDGE('',*,*,#8132,.F.);
#11585=ORIENTED_EDGE('',*,*,#8173,.F.);
#11586=ORIENTED_EDGE('',*,*,#8176,.F.);
#11587=ORIENTED_EDGE('',*,*,#8178,.F.);
#11588=ORIENTED_EDGE('',*,*,#8180,.F.);
#11589=ORIENTED_EDGE('',*,*,#8182,.F.);
#11590=ORIENTED_EDGE('',*,*,#8185,.F.);
#11591=ORIENTED_EDGE('',*,*,#8188,.F.);
#11592=ORIENTED_EDGE('',*,*,#8190,.F.);
#11593=ORIENTED_EDGE('',*,*,#8200,.T.);
#11594=ORIENTED_EDGE('',*,*,#8201,.F.);
#11595=ORIENTED_EDGE('',*,*,#8102,.T.);
#11596=ORIENTED_EDGE('',*,*,#8112,.T.);
#11597=ORIENTED_EDGE('',*,*,#8108,.T.);
#11598=ORIENTED_EDGE('',*,*,#8202,.F.);
#11599=ORIENTED_EDGE('',*,*,#8142,.T.);
#11600=ORIENTED_EDGE('',*,*,#8097,.T.);
#11601=ORIENTED_EDGE('',*,*,#8202,.T.);
#11602=ORIENTED_EDGE('',*,*,#8107,.T.);
#11603=ORIENTED_EDGE('',*,*,#8203,.T.);
#11604=ORIENTED_EDGE('',*,*,#8143,.T.);
#11605=ORIENTED_EDGE('',*,*,#8204,.T.);
#11606=ORIENTED_EDGE('',*,*,#8193,.T.);
#11607=ORIENTED_EDGE('',*,*,#8205,.T.);
#11608=ORIENTED_EDGE('',*,*,#8105,.T.);
#11609=ORIENTED_EDGE('',*,*,#8205,.F.);
#11610=ORIENTED_EDGE('',*,*,#8192,.T.);
#11611=ORIENTED_EDGE('',*,*,#8203,.F.);
#11612=ORIENTED_EDGE('',*,*,#8106,.T.);
#11613=ORIENTED_EDGE('',*,*,#8201,.T.);
#11614=ORIENTED_EDGE('',*,*,#8206,.T.);
#11615=ORIENTED_EDGE('',*,*,#8207,.T.);
#11616=ORIENTED_EDGE('',*,*,#8103,.T.);
#11617=ORIENTED_EDGE('',*,*,#8207,.F.);
#11618=ORIENTED_EDGE('',*,*,#8194,.T.);
#11619=ORIENTED_EDGE('',*,*,#8204,.F.);
#11620=ORIENTED_EDGE('',*,*,#8104,.T.);
#11621=ORIENTED_EDGE('',*,*,#8206,.F.);
#11622=ORIENTED_EDGE('',*,*,#8200,.F.);
#11623=ORIENTED_EDGE('',*,*,#8111,.T.);
#11624=ORIENTED_EDGE('',*,*,#8208,.F.);
#11625=ORIENTED_EDGE('',*,*,#8209,.F.);
#11626=ORIENTED_EDGE('',*,*,#8195,.T.);
#11627=ORIENTED_EDGE('',*,*,#8210,.T.);
#11628=ORIENTED_EDGE('',*,*,#8211,.F.);
#11629=ORIENTED_EDGE('',*,*,#8114,.T.);
#11630=ORIENTED_EDGE('',*,*,#8212,.T.);
#11631=ORIENTED_EDGE('',*,*,#8120,.T.);
#11632=ORIENTED_EDGE('',*,*,#8213,.F.);
#11633=ORIENTED_EDGE('',*,*,#8208,.T.);
#11634=ORIENTED_EDGE('',*,*,#8110,.T.);
#11635=ORIENTED_EDGE('',*,*,#8213,.T.);
#11636=ORIENTED_EDGE('',*,*,#8119,.T.);
#11637=ORIENTED_EDGE('',*,*,#8214,.T.);
#11638=ORIENTED_EDGE('',*,*,#8209,.T.);
#11639=ORIENTED_EDGE('',*,*,#8215,.T.);
#11640=ORIENTED_EDGE('',*,*,#8197,.T.);
#11641=ORIENTED_EDGE('',*,*,#8216,.T.);
#11642=ORIENTED_EDGE('',*,*,#8117,.T.);
#11643=ORIENTED_EDGE('',*,*,#8216,.F.);
#11644=ORIENTED_EDGE('',*,*,#8196,.T.);
#11645=ORIENTED_EDGE('',*,*,#8214,.F.);
#11646=ORIENTED_EDGE('',*,*,#8118,.T.);
#11647=ORIENTED_EDGE('',*,*,#8211,.T.);
#11648=ORIENTED_EDGE('',*,*,#8217,.T.);
#11649=ORIENTED_EDGE('',*,*,#8218,.T.);
#11650=ORIENTED_EDGE('',*,*,#8115,.T.);
#11651=ORIENTED_EDGE('',*,*,#8218,.F.);
#11652=ORIENTED_EDGE('',*,*,#8198,.T.);
#11653=ORIENTED_EDGE('',*,*,#8215,.F.);
#11654=ORIENTED_EDGE('',*,*,#8116,.T.);
#11655=ORIENTED_EDGE('',*,*,#8156,.F.);
#11656=ORIENTED_EDGE('',*,*,#8199,.T.);
#11657=ORIENTED_EDGE('',*,*,#8217,.F.);
#11658=ORIENTED_EDGE('',*,*,#8210,.F.);
#11659=ORIENTED_EDGE('',*,*,#8219,.T.);
#11660=ORIENTED_EDGE('',*,*,#8152,.F.);
#11661=ORIENTED_EDGE('',*,*,#8095,.F.);
#11662=ORIENTED_EDGE('',*,*,#8171,.T.);
#11663=ORIENTED_EDGE('',*,*,#8153,.F.);
#11664=ORIENTED_EDGE('',*,*,#8219,.F.);
#11665=ORIENTED_EDGE('',*,*,#8212,.F.);
#11666=ORIENTED_EDGE('',*,*,#8113,.F.);
#11667=ORIENTED_EDGE('',*,*,#8017,.F.);
#11668=ORIENTED_EDGE('',*,*,#8028,.T.);
#11669=ORIENTED_EDGE('',*,*,#8191,.F.);
#11670=ORIENTED_EDGE('',*,*,#8220,.F.);
#11671=ORIENTED_EDGE('',*,*,#8020,.F.);
#11672=ORIENTED_EDGE('',*,*,#8220,.T.);
#11673=ORIENTED_EDGE('',*,*,#8189,.F.);
#11674=ORIENTED_EDGE('',*,*,#8221,.F.);
#11675=ORIENTED_EDGE('',*,*,#8023,.F.);
#11676=ORIENTED_EDGE('',*,*,#8221,.T.);
#11677=ORIENTED_EDGE('',*,*,#8186,.F.);
#11678=ORIENTED_EDGE('',*,*,#8222,.F.);
#11679=ORIENTED_EDGE('',*,*,#8025,.F.);
#11680=ORIENTED_EDGE('',*,*,#8222,.T.);
#11681=ORIENTED_EDGE('',*,*,#8183,.F.);
#11682=ORIENTED_EDGE('',*,*,#8033,.F.);
#11683=ORIENTED_EDGE('',*,*,#8061,.F.);
#11684=ORIENTED_EDGE('',*,*,#8223,.T.);
#11685=ORIENTED_EDGE('',*,*,#8039,.T.);
#11686=ORIENTED_EDGE('',*,*,#8224,.F.);
#11687=ORIENTED_EDGE('',*,*,#8064,.F.);
#11688=ORIENTED_EDGE('',*,*,#8224,.T.);
#11689=ORIENTED_EDGE('',*,*,#8038,.T.);
#11690=ORIENTED_EDGE('',*,*,#8225,.F.);
#11691=ORIENTED_EDGE('',*,*,#8066,.F.);
#11692=ORIENTED_EDGE('',*,*,#8225,.T.);
#11693=ORIENTED_EDGE('',*,*,#8037,.T.);
#11694=ORIENTED_EDGE('',*,*,#8071,.F.);
#11695=ORIENTED_EDGE('',*,*,#8058,.F.);
#11696=ORIENTED_EDGE('',*,*,#8068,.T.);
#11697=ORIENTED_EDGE('',*,*,#8040,.T.);
#11698=ORIENTED_EDGE('',*,*,#8223,.F.);
#12850=PLANE('',#14691);
#12851=PLANE('',#14695);
#12852=PLANE('',#14699);
#12853=PLANE('',#14703);
#12854=PLANE('',#14709);
#12855=PLANE('',#14712);
#12856=PLANE('',#14713);
#12857=PLANE('',#14721);
#12858=PLANE('',#14725);
#12859=PLANE('',#14729);
#12860=PLANE('',#14733);
#12861=PLANE('',#14734);
#12862=PLANE('',#14736);
#12863=PLANE('',#14738);
#12864=PLANE('',#14745);
#12865=PLANE('',#14748);
#12866=PLANE('',#14751);
#12867=PLANE('',#14754);
#12868=PLANE('',#14755);
#12869=PLANE('',#14758);
#12870=PLANE('',#14770);
#12871=PLANE('',#14774);
#12872=PLANE('',#14777);
#12873=PLANE('',#14781);
#12874=PLANE('',#14785);
#12875=PLANE('',#14786);
#12876=PLANE('',#14793);
#12877=PLANE('',#14794);
#12878=PLANE('',#14796);
#12879=PLANE('',#14798);
#12880=PLANE('',#14800);
#13538=ADVANCED_FACE('',(#1775),#12850,.T.);
#13539=ADVANCED_FACE('',(#1776),#1208,.F.);
#13540=ADVANCED_FACE('',(#1777),#12851,.T.);
#13541=ADVANCED_FACE('',(#1778),#1209,.F.);
#13542=ADVANCED_FACE('',(#1779),#12852,.T.);
#13543=ADVANCED_FACE('',(#1780),#1210,.F.);
#13544=ADVANCED_FACE('',(#1781),#12853,.T.);
#13545=ADVANCED_FACE('',(#1782),#1211,.F.);
#13546=ADVANCED_FACE('',(#1783),#744,.F.);
#13547=ADVANCED_FACE('',(#1784),#12854,.T.);
#13548=ADVANCED_FACE('',(#1785),#745,.F.);
#13549=ADVANCED_FACE('',(#1786),#12855,.T.);
#13550=ADVANCED_FACE('',(#1787,#642),#12856,.T.);
#13551=ADVANCED_FACE('',(#1788),#1212,.F.);
#13552=ADVANCED_FACE('',(#1789),#12857,.T.);
#13553=ADVANCED_FACE('',(#1790),#1213,.F.);
#13554=ADVANCED_FACE('',(#1791),#12858,.T.);
#13555=ADVANCED_FACE('',(#1792),#1214,.F.);
#13556=ADVANCED_FACE('',(#1793),#12859,.T.);
#13557=ADVANCED_FACE('',(#1794),#1215,.F.);
#13558=ADVANCED_FACE('',(#1795),#12860,.T.);
#13559=ADVANCED_FACE('',(#1796),#12861,.T.);
#13560=ADVANCED_FACE('',(#1797),#746,.F.);
#13561=ADVANCED_FACE('',(#1798),#12862,.T.);
#13562=ADVANCED_FACE('',(#1799),#747,.F.);
#13563=ADVANCED_FACE('',(#1800,#643),#12863,.T.);
#13564=ADVANCED_FACE('',(#1801),#1216,.T.);
#13565=ADVANCED_FACE('',(#1802),#12864,.T.);
#13566=ADVANCED_FACE('',(#1803),#1217,.T.);
#13567=ADVANCED_FACE('',(#1804),#12865,.T.);
#13568=ADVANCED_FACE('',(#1805),#1218,.T.);
#13569=ADVANCED_FACE('',(#1806),#12866,.T.);
#13570=ADVANCED_FACE('',(#1807),#1219,.T.);
#13571=ADVANCED_FACE('',(#1808),#12867,.T.);
#13572=ADVANCED_FACE('',(#1809),#12868,.T.);
#13573=ADVANCED_FACE('',(#1810),#748,.T.);
#13574=ADVANCED_FACE('',(#1811),#12869,.T.);
#13575=ADVANCED_FACE('',(#1812),#749,.T.);
#13576=ADVANCED_FACE('',(#1813),#487,.T.);
#13577=ADVANCED_FACE('',(#1814),#488,.T.);
#13578=ADVANCED_FACE('',(#1815),#489,.T.);
#13579=ADVANCED_FACE('',(#1816),#1220,.T.);
#13580=ADVANCED_FACE('',(#1817),#490,.T.);
#13581=ADVANCED_FACE('',(#1818),#491,.T.);
#13582=ADVANCED_FACE('',(#1819),#492,.T.);
#13583=ADVANCED_FACE('',(#1820),#750,.T.);
#13584=ADVANCED_FACE('',(#1821),#751,.T.);
#13585=ADVANCED_FACE('',(#1822),#493,.T.);
#13586=ADVANCED_FACE('',(#1823),#494,.T.);
#13587=ADVANCED_FACE('',(#1824),#495,.T.);
#13588=ADVANCED_FACE('',(#1825),#1221,.T.);
#13589=ADVANCED_FACE('',(#1826),#496,.T.);
#13590=ADVANCED_FACE('',(#1827),#497,.T.);
#13591=ADVANCED_FACE('',(#1828),#498,.T.);
#13592=ADVANCED_FACE('',(#1829),#752,.T.);
#13593=ADVANCED_FACE('',(#1830),#12870,.T.);
#13594=ADVANCED_FACE('',(#1831),#753,.T.);
#13595=ADVANCED_FACE('',(#1832),#1222,.F.);
#13596=ADVANCED_FACE('',(#1833),#12871,.T.);
#13597=ADVANCED_FACE('',(#1834),#1223,.F.);
#13598=ADVANCED_FACE('',(#1835),#12872,.T.);
#13599=ADVANCED_FACE('',(#1836),#1224,.F.);
#13600=ADVANCED_FACE('',(#1837),#12873,.T.);
#13601=ADVANCED_FACE('',(#1838),#1225,.F.);
#13602=ADVANCED_FACE('',(#1839),#12874,.T.);
#13603=ADVANCED_FACE('',(#1840,#644),#12875,.F.);
#13604=ADVANCED_FACE('',(#1841),#499,.T.);
#13605=ADVANCED_FACE('',(#1842),#500,.T.);
#13606=ADVANCED_FACE('',(#1843),#501,.T.);
#13607=ADVANCED_FACE('',(#1844),#1226,.T.);
#13608=ADVANCED_FACE('',(#1845),#502,.T.);
#13609=ADVANCED_FACE('',(#1846),#503,.T.);
#13610=ADVANCED_FACE('',(#1847),#504,.T.);
#13611=ADVANCED_FACE('',(#1848),#754,.T.);
#13612=ADVANCED_FACE('',(#1849),#505,.T.);
#13613=ADVANCED_FACE('',(#1850),#506,.T.);
#13614=ADVANCED_FACE('',(#1851),#507,.T.);
#13615=ADVANCED_FACE('',(#1852),#1227,.T.);
#13616=ADVANCED_FACE('',(#1853),#508,.T.);
#13617=ADVANCED_FACE('',(#1854),#509,.T.);
#13618=ADVANCED_FACE('',(#1855),#510,.T.);
#13619=ADVANCED_FACE('',(#1856),#755,.T.);
#13620=ADVANCED_FACE('',(#1857),#12876,.T.);
#13621=ADVANCED_FACE('',(#1858),#12877,.T.);
#13622=ADVANCED_FACE('',(#1859),#756,.F.);
#13623=ADVANCED_FACE('',(#1860),#12878,.T.);
#13624=ADVANCED_FACE('',(#1861),#757,.F.);
#13625=ADVANCED_FACE('',(#1862),#12879,.T.);
#13626=ADVANCED_FACE('',(#1863),#758,.F.);
#13627=ADVANCED_FACE('',(#1864),#12880,.T.);
#13628=ADVANCED_FACE('',(#1865),#759,.F.);
#13815=CLOSED_SHELL('',(#13538,#13539,#13540,#13541,#13542,#13543,#13544,
#13545,#13546,#13547,#13548,#13549,#13550,#13551,#13552,#13553,#13554,#13555,
#13556,#13557,#13558,#13559,#13560,#13561,#13562,#13563,#13564,#13565,#13566,
#13567,#13568,#13569,#13570,#13571,#13572,#13573,#13574,#13575,#13576,#13577,
#13578,#13579,#13580,#13581,#13582,#13583,#13584,#13585,#13586,#13587,#13588,
#13589,#13590,#13591,#13592,#13593,#13594,#13595,#13596,#13597,#13598,#13599,
#13600,#13601,#13602,#13603,#13604,#13605,#13606,#13607,#13608,#13609,#13610,
#13611,#13612,#13613,#13614,#13615,#13616,#13617,#13618,#13619,#13620,#13621,
#13622,#13623,#13624,#13625,#13626,#13627,#13628));
#14690=AXIS2_PLACEMENT_3D('',#26844,#17260,#17261);
#14691=AXIS2_PLACEMENT_3D('',#26845,#17262,#17263);
#14692=AXIS2_PLACEMENT_3D('',#26854,#17268,#17269);
#14693=AXIS2_PLACEMENT_3D('',#26858,#17271,#17272);
#14694=AXIS2_PLACEMENT_3D('',#26859,#17273,#17274);
#14695=AXIS2_PLACEMENT_3D('',#26860,#17275,#17276);
#14696=AXIS2_PLACEMENT_3D('',#26866,#17280,#17281);
#14697=AXIS2_PLACEMENT_3D('',#26870,#17283,#17284);
#14698=AXIS2_PLACEMENT_3D('',#26871,#17285,#17286);
#14699=AXIS2_PLACEMENT_3D('',#26872,#17287,#17288);
#14700=AXIS2_PLACEMENT_3D('',#26878,#17292,#17293);
#14701=AXIS2_PLACEMENT_3D('',#26882,#17295,#17296);
#14702=AXIS2_PLACEMENT_3D('',#26883,#17297,#17298);
#14703=AXIS2_PLACEMENT_3D('',#26884,#17299,#17300);
#14704=AXIS2_PLACEMENT_3D('',#26890,#17304,#17305);
#14705=AXIS2_PLACEMENT_3D('',#26891,#17306,#17307);
#14706=AXIS2_PLACEMENT_3D('',#26892,#17308,#17309);
#14707=AXIS2_PLACEMENT_3D('',#26893,#17310,#17311);
#14708=AXIS2_PLACEMENT_3D('',#26897,#17313,#17314);
#14709=AXIS2_PLACEMENT_3D('',#26899,#17316,#17317);
#14710=AXIS2_PLACEMENT_3D('',#26903,#17320,#17321);
#14711=AXIS2_PLACEMENT_3D('',#26906,#17323,#17324);
#14712=AXIS2_PLACEMENT_3D('',#26907,#17325,#17326);
#14713=AXIS2_PLACEMENT_3D('',#26911,#17329,#17330);
#14714=AXIS2_PLACEMENT_3D('',#26916,#17332,#17333);
#14715=AXIS2_PLACEMENT_3D('',#26920,#17335,#17336);
#14716=AXIS2_PLACEMENT_3D('',#26924,#17338,#17339);
#14717=AXIS2_PLACEMENT_3D('',#26927,#17341,#17342);
#14718=AXIS2_PLACEMENT_3D('',#26928,#17343,#17344);
#14719=AXIS2_PLACEMENT_3D('',#26933,#17346,#17347);
#14720=AXIS2_PLACEMENT_3D('',#26936,#17349,#17350);
#14721=AXIS2_PLACEMENT_3D('',#26937,#17351,#17352);
#14722=AXIS2_PLACEMENT_3D('',#26943,#17356,#17357);
#14723=AXIS2_PLACEMENT_3D('',#26947,#17359,#17360);
#14724=AXIS2_PLACEMENT_3D('',#26948,#17361,#17362);
#14725=AXIS2_PLACEMENT_3D('',#26949,#17363,#17364);
#14726=AXIS2_PLACEMENT_3D('',#26955,#17368,#17369);
#14727=AXIS2_PLACEMENT_3D('',#26959,#17371,#17372);
#14728=AXIS2_PLACEMENT_3D('',#26960,#17373,#17374);
#14729=AXIS2_PLACEMENT_3D('',#26961,#17375,#17376);
#14730=AXIS2_PLACEMENT_3D('',#26967,#17380,#17381);
#14731=AXIS2_PLACEMENT_3D('',#26971,#17383,#17384);
#14732=AXIS2_PLACEMENT_3D('',#26972,#17385,#17386);
#14733=AXIS2_PLACEMENT_3D('',#26973,#17387,#17388);
#14734=AXIS2_PLACEMENT_3D('',#26976,#17391,#17392);
#14735=AXIS2_PLACEMENT_3D('',#26979,#17395,#17396);
#14736=AXIS2_PLACEMENT_3D('',#26981,#17398,#17399);
#14737=AXIS2_PLACEMENT_3D('',#26983,#17401,#17402);
#14738=AXIS2_PLACEMENT_3D('',#26985,#17404,#17405);
#14739=AXIS2_PLACEMENT_3D('',#26988,#17406,#17407);
#14740=AXIS2_PLACEMENT_3D('',#26992,#17409,#17410);
#14741=AXIS2_PLACEMENT_3D('',#26996,#17412,#17413);
#14742=AXIS2_PLACEMENT_3D('',#27000,#17415,#17416);
#14743=AXIS2_PLACEMENT_3D('',#27002,#17418,#17419);
#14744=AXIS2_PLACEMENT_3D('',#27007,#17422,#17423);
#14745=AXIS2_PLACEMENT_3D('',#27008,#17424,#17425);
#14746=AXIS2_PLACEMENT_3D('',#27012,#17428,#17429);
#14747=AXIS2_PLACEMENT_3D('',#27015,#17431,#17432);
#14748=AXIS2_PLACEMENT_3D('',#27016,#17433,#17434);
#14749=AXIS2_PLACEMENT_3D('',#27020,#17437,#17438);
#14750=AXIS2_PLACEMENT_3D('',#27023,#17440,#17441);
#14751=AXIS2_PLACEMENT_3D('',#27024,#17442,#17443);
#14752=AXIS2_PLACEMENT_3D('',#27028,#17446,#17447);
#14753=AXIS2_PLACEMENT_3D('',#27031,#17449,#17450);
#14754=AXIS2_PLACEMENT_3D('',#27032,#17451,#17452);
#14755=AXIS2_PLACEMENT_3D('',#27034,#17454,#17455);
#14756=AXIS2_PLACEMENT_3D('',#27044,#17461,#17462);
#14757=AXIS2_PLACEMENT_3D('',#27127,#17464,#17465);
#14758=AXIS2_PLACEMENT_3D('',#27208,#17466,#17467);
#14759=AXIS2_PLACEMENT_3D('',#27216,#17472,#17473);
#14760=AXIS2_PLACEMENT_3D('',#27300,#17475,#17476);
#14761=AXIS2_PLACEMENT_3D('',#27835,#17479,#17480);
#14762=AXIS2_PLACEMENT_3D('',#27840,#17482,#17483);
#14763=AXIS2_PLACEMENT_3D('',#27843,#17485,#17486);
#14764=AXIS2_PLACEMENT_3D('',#27943,#17488,#17489);
#14765=AXIS2_PLACEMENT_3D('',#28051,#17491,#17492);
#14766=AXIS2_PLACEMENT_3D('',#28530,#17497,#17498);
#14767=AXIS2_PLACEMENT_3D('',#28535,#17500,#17501);
#14768=AXIS2_PLACEMENT_3D('',#28538,#17503,#17504);
#14769=AXIS2_PLACEMENT_3D('',#28620,#17506,#17507);
#14770=AXIS2_PLACEMENT_3D('',#28623,#17510,#17511);
#14771=AXIS2_PLACEMENT_3D('',#28625,#17513,#17514);
#14772=AXIS2_PLACEMENT_3D('',#28627,#17516,#17517);
#14773=AXIS2_PLACEMENT_3D('',#28631,#17519,#17520);
#14774=AXIS2_PLACEMENT_3D('',#28633,#17522,#17523);
#14775=AXIS2_PLACEMENT_3D('',#28637,#17526,#17527);
#14776=AXIS2_PLACEMENT_3D('',#28640,#17529,#17530);
#14777=AXIS2_PLACEMENT_3D('',#28641,#17531,#17532);
#14778=AXIS2_PLACEMENT_3D('',#28645,#17535,#17536);
#14779=AXIS2_PLACEMENT_3D('',#28649,#17538,#17539);
#14780=AXIS2_PLACEMENT_3D('',#28650,#17540,#17541);
#14781=AXIS2_PLACEMENT_3D('',#28651,#17542,#17543);
#14782=AXIS2_PLACEMENT_3D('',#28657,#17547,#17548);
#14783=AXIS2_PLACEMENT_3D('',#28661,#17550,#17551);
#14784=AXIS2_PLACEMENT_3D('',#28662,#17552,#17553);
#14785=AXIS2_PLACEMENT_3D('',#28663,#17554,#17555);
#14786=AXIS2_PLACEMENT_3D('',#28666,#17558,#17559);
#14787=AXIS2_PLACEMENT_3D('',#28673,#17560,#17561);
#14788=AXIS2_PLACEMENT_3D('',#28687,#17563,#17564);
#14789=AXIS2_PLACEMENT_3D('',#28909,#17567,#17568);
#14790=AXIS2_PLACEMENT_3D('',#28970,#17572,#17573);
#14791=AXIS2_PLACEMENT_3D('',#29283,#17576,#17577);
#14792=AXIS2_PLACEMENT_3D('',#29349,#17581,#17582);
#14793=AXIS2_PLACEMENT_3D('',#29351,#17584,#17585);
#14794=AXIS2_PLACEMENT_3D('',#29352,#17586,#17587);
#14795=AXIS2_PLACEMENT_3D('',#29354,#17589,#17590);
#14796=AXIS2_PLACEMENT_3D('',#29356,#17592,#17593);
#14797=AXIS2_PLACEMENT_3D('',#29358,#17595,#17596);
#14798=AXIS2_PLACEMENT_3D('',#29359,#17597,#17598);
#14799=AXIS2_PLACEMENT_3D('',#29362,#17601,#17602);
#14800=AXIS2_PLACEMENT_3D('',#29364,#17604,#17605);
#14801=AXIS2_PLACEMENT_3D('',#29365,#17606,#17607);
#17260=DIRECTION('axis',(0.,0.,1.));
#17261=DIRECTION('refdir',(1.,0.,0.));
#17262=DIRECTION('center_axis',(0.707106781186545,0.70710678118655,0.));
#17263=DIRECTION('ref_axis',(0.,0.,-1.));
#17264=DIRECTION('',(-0.70710678118655,0.707106781186545,0.));
#17265=DIRECTION('',(0.,0.,1.));
#17266=DIRECTION('',(0.70710678118655,-0.707106781186545,-7.85046229341888E-16));
#17267=DIRECTION('',(0.,0.,-1.));
#17268=DIRECTION('center_axis',(0.,1.,0.));
#17269=DIRECTION('ref_axis',(-3.96508223080413E-16,0.,-1.));
#17270=DIRECTION('',(-3.92523114670943E-16,0.707106781186544,-0.707106781186551));
#17271=DIRECTION('center_axis',(0.,1.,0.));
#17272=DIRECTION('ref_axis',(-3.96508223080413E-16,0.,-1.));
#17273=DIRECTION('center_axis',(0.,-1.,0.));
#17274=DIRECTION('ref_axis',(-3.96508223080413E-16,0.,-1.));
#17275=DIRECTION('center_axis',(0.,0.707106781186549,0.707106781186546));
#17276=DIRECTION('ref_axis',(1.,0.,0.));
#17277=DIRECTION('',(0.,0.707106781186546,-0.707106781186549));
#17278=DIRECTION('',(-1.,0.,0.));
#17279=DIRECTION('',(1.,0.,0.));
#17280=DIRECTION('center_axis',(0.,1.,0.));
#17281=DIRECTION('ref_axis',(1.,0.,-9.51619735392991E-16));
#17282=DIRECTION('',(0.707106781186548,0.707106781186548,-7.8504622934189E-16));
#17283=DIRECTION('center_axis',(0.,1.,0.));
#17284=DIRECTION('ref_axis',(1.,0.,-9.51619735392991E-16));
#17285=DIRECTION('center_axis',(0.,-1.,0.));
#17286=DIRECTION('ref_axis',(1.,0.,-9.51619735392991E-16));
#17287=DIRECTION('center_axis',(-0.707106781186548,0.707106781186548,0.));
#17288=DIRECTION('ref_axis',(0.,0.,1.));
#17289=DIRECTION('',(0.707106781186548,0.707106781186548,0.));
#17290=DIRECTION('',(0.,0.,-1.));
#17291=DIRECTION('',(0.,0.,1.));
#17292=DIRECTION('center_axis',(0.,1.,0.));
#17293=DIRECTION('ref_axis',(6.3441315692866E-16,0.,1.));
#17294=DIRECTION('',(0.,0.707106781186546,0.707106781186549));
#17295=DIRECTION('center_axis',(0.,1.,0.));
#17296=DIRECTION('ref_axis',(6.3441315692866E-16,0.,1.));
#17297=DIRECTION('center_axis',(0.,-1.,0.));
#17298=DIRECTION('ref_axis',(6.3441315692866E-16,0.,1.));
#17299=DIRECTION('center_axis',(0.,0.707106781186549,-0.707106781186546));
#17300=DIRECTION('ref_axis',(-1.,0.,0.));
#17301=DIRECTION('',(3.92523114670944E-16,0.707106781186546,0.707106781186549));
#17302=DIRECTION('',(1.,0.,0.));
#17303=DIRECTION('',(-1.,0.,0.));
#17304=DIRECTION('center_axis',(0.,1.,0.));
#17305=DIRECTION('ref_axis',(-1.,0.,3.1720657846433E-16));
#17306=DIRECTION('center_axis',(0.,1.,0.));
#17307=DIRECTION('ref_axis',(-1.,0.,3.1720657846433E-16));
#17308=DIRECTION('center_axis',(0.,-1.,0.));
#17309=DIRECTION('ref_axis',(-1.,0.,3.1720657846433E-16));
#17310=DIRECTION('center_axis',(0.,-1.,0.));
#17311=DIRECTION('ref_axis',(1.,0.,-9.51619735392991E-16));
#17312=DIRECTION('',(0.,-1.,0.));
#17313=DIRECTION('center_axis',(0.,1.,0.));
#17314=DIRECTION('ref_axis',(1.,0.,-9.51619735392991E-16));
#17315=DIRECTION('',(0.,-1.,0.));
#17316=DIRECTION('center_axis',(0.,0.,1.));
#17317=DIRECTION('ref_axis',(-1.,0.,0.));
#17318=DIRECTION('',(0.,-1.,0.));
#17319=DIRECTION('',(-1.,0.,0.));
#17320=DIRECTION('center_axis',(0.,-1.,0.));
#17321=DIRECTION('ref_axis',(-3.96508223080413E-16,0.,-1.));
#17322=DIRECTION('',(0.,-1.,0.));
#17323=DIRECTION('center_axis',(0.,1.,0.));
#17324=DIRECTION('ref_axis',(-3.96508223080413E-16,0.,-1.));
#17325=DIRECTION('center_axis',(1.,0.,0.));
#17326=DIRECTION('ref_axis',(0.,0.,1.));
#17327=DIRECTION('',(0.,-1.,0.));
#17328=DIRECTION('',(0.,0.,1.));
#17329=DIRECTION('center_axis',(0.,1.,0.));
#17330=DIRECTION('ref_axis',(1.,0.,0.));
#17331=DIRECTION('',(0.,0.,1.));
#17332=DIRECTION('center_axis',(0.,-1.,0.));
#17333=DIRECTION('ref_axis',(1.,0.,0.));
#17334=DIRECTION('',(1.,0.,0.));
#17335=DIRECTION('center_axis',(0.,-1.,0.));
#17336=DIRECTION('ref_axis',(-6.5658350918692E-16,0.,-1.));
#17337=DIRECTION('',(0.,0.,-1.));
#17338=DIRECTION('center_axis',(0.,-1.,0.));
#17339=DIRECTION('ref_axis',(-1.,0.,5.96894099260836E-16));
#17340=DIRECTION('',(-1.,0.,0.));
#17341=DIRECTION('center_axis',(0.,-1.,0.));
#17342=DIRECTION('ref_axis',(4.7751527940867E-16,0.,1.));
#17343=DIRECTION('center_axis',(0.,1.,0.));
#17344=DIRECTION('ref_axis',(1.,0.,0.));
#17345=DIRECTION('',(0.707106781186548,0.707106781186548,0.));
#17346=DIRECTION('center_axis',(0.,1.,0.));
#17347=DIRECTION('ref_axis',(1.,0.,0.));
#17348=DIRECTION('',(0.,-0.707106781186544,0.707106781186551));
#17349=DIRECTION('center_axis',(0.,-1.,0.));
#17350=DIRECTION('ref_axis',(1.,0.,0.));
#17351=DIRECTION('center_axis',(-0.707106781186548,0.707106781186548,0.));
#17352=DIRECTION('ref_axis',(0.,0.,1.));
#17353=DIRECTION('',(0.707106781186551,0.707106781186544,0.));
#17354=DIRECTION('',(0.,0.,-1.));
#17355=DIRECTION('',(0.,0.,1.));
#17356=DIRECTION('center_axis',(0.,1.,0.));
#17357=DIRECTION('ref_axis',(4.7751527940867E-16,0.,1.));
#17358=DIRECTION('',(0.,0.707106781186548,0.707106781186548));
#17359=DIRECTION('center_axis',(0.,1.,0.));
#17360=DIRECTION('ref_axis',(4.7751527940867E-16,0.,1.));
#17361=DIRECTION('center_axis',(0.,-1.,0.));
#17362=DIRECTION('ref_axis',(4.7751527940867E-16,0.,1.));
#17363=DIRECTION('center_axis',(0.,0.707106781186549,-0.707106781186546));
#17364=DIRECTION('ref_axis',(-1.,0.,0.));
#17365=DIRECTION('',(-3.92523114670944E-16,0.707106781186546,0.707106781186549));
#17366=DIRECTION('',(1.,0.,0.));
#17367=DIRECTION('',(-1.,0.,0.));
#17368=DIRECTION('center_axis',(0.,1.,0.));
#17369=DIRECTION('ref_axis',(-1.,0.,5.96894099260837E-16));
#17370=DIRECTION('',(-0.707106781186548,0.707106781186547,7.85046229341889E-16));
#17371=DIRECTION('center_axis',(0.,1.,0.));
#17372=DIRECTION('ref_axis',(-1.,0.,5.96894099260836E-16));
#17373=DIRECTION('center_axis',(0.,-1.,0.));
#17374=DIRECTION('ref_axis',(-1.,0.,5.96894099260836E-16));
#17375=DIRECTION('center_axis',(0.707106781186547,0.707106781186548,0.));
#17376=DIRECTION('ref_axis',(0.,0.,-1.));
#17377=DIRECTION('',(-0.707106781186548,0.707106781186547,0.));
#17378=DIRECTION('',(0.,0.,1.));
#17379=DIRECTION('',(0.,0.,-1.));
#17380=DIRECTION('center_axis',(0.,1.,0.));
#17381=DIRECTION('ref_axis',(-6.5658350918692E-16,0.,-1.));
#17382=DIRECTION('',(-3.92523114670945E-16,0.707106781186548,-0.707106781186548));
#17383=DIRECTION('center_axis',(0.,1.,0.));
#17384=DIRECTION('ref_axis',(-6.5658350918692E-16,0.,-1.));
#17385=DIRECTION('center_axis',(0.,-1.,0.));
#17386=DIRECTION('ref_axis',(-6.5658350918692E-16,0.,-1.));
#17387=DIRECTION('center_axis',(0.,0.707106781186549,0.707106781186546));
#17388=DIRECTION('ref_axis',(1.,0.,0.));
#17389=DIRECTION('',(-1.,0.,0.));
#17390=DIRECTION('',(1.,0.,0.));
#17391=DIRECTION('center_axis',(0.,0.,-1.));
#17392=DIRECTION('ref_axis',(1.,0.,0.));
#17393=DIRECTION('',(0.,-1.,0.));
#17394=DIRECTION('',(0.,-1.,0.));
#17395=DIRECTION('center_axis',(0.,-1.,0.));
#17396=DIRECTION('ref_axis',(4.7751527940867E-16,0.,1.));
#17397=DIRECTION('',(0.,-1.,0.));
#17398=DIRECTION('center_axis',(-1.,0.,0.));
#17399=DIRECTION('ref_axis',(0.,0.,-1.));
#17400=DIRECTION('',(0.,-1.,0.));
#17401=DIRECTION('center_axis',(0.,-1.,0.));
#17402=DIRECTION('ref_axis',(1.,0.,0.));
#17403=DIRECTION('',(0.,-1.,0.));
#17404=DIRECTION('center_axis',(0.,1.,0.));
#17405=DIRECTION('ref_axis',(1.,0.,0.));
#17406=DIRECTION('center_axis',(0.,-1.,0.));
#17407=DIRECTION('ref_axis',(1.26882631385732E-15,0.,1.));
#17408=DIRECTION('',(0.,0.,1.));
#17409=DIRECTION('center_axis',(0.,-1.,0.));
#17410=DIRECTION('ref_axis',(1.,0.,-1.26882631385732E-15));
#17411=DIRECTION('',(1.,0.,0.));
#17412=DIRECTION('center_axis',(0.,-1.,0.));
#17413=DIRECTION('ref_axis',(-9.51619735392991E-16,0.,-1.));
#17414=DIRECTION('',(0.,0.,-1.));
#17415=DIRECTION('center_axis',(0.,-1.,0.));
#17416=DIRECTION('ref_axis',(-1.,0.,6.3441315692866E-16));
#17417=DIRECTION('',(-1.,0.,0.));
#17418=DIRECTION('center_axis',(0.,-1.,0.));
#17419=DIRECTION('ref_axis',(1.26882631385732E-15,0.,1.));
#17420=DIRECTION('',(-0.707106781186548,0.707106781186548,0.));
#17421=DIRECTION('',(0.,-0.707106781186548,0.707106781186548));
#17422=DIRECTION('center_axis',(0.,1.,0.));
#17423=DIRECTION('ref_axis',(1.26882631385732E-15,0.,1.));
#17424=DIRECTION('center_axis',(0.707106781186548,0.707106781186548,0.));
#17425=DIRECTION('ref_axis',(0.,0.,-1.));
#17426=DIRECTION('',(0.,0.,-1.));
#17427=DIRECTION('',(-0.707106781186548,0.707106781186548,0.));
#17428=DIRECTION('center_axis',(0.,-1.,0.));
#17429=DIRECTION('ref_axis',(1.,0.,-1.26882631385732E-15));
#17430=DIRECTION('',(0.,0.707106781186548,0.707106781186548));
#17431=DIRECTION('center_axis',(0.,1.,0.));
#17432=DIRECTION('ref_axis',(1.,0.,-1.26882631385732E-15));
#17433=DIRECTION('center_axis',(0.,0.707106781186548,-0.707106781186548));
#17434=DIRECTION('ref_axis',(-1.,0.,0.));
#17435=DIRECTION('',(-1.,0.,0.));
#17436=DIRECTION('',(1.57009245868378E-15,0.707106781186548,0.707106781186548));
#17437=DIRECTION('center_axis',(0.,-1.,0.));
#17438=DIRECTION('ref_axis',(-9.5161973539299E-16,0.,-1.));
#17439=DIRECTION('',(0.707106781186551,0.707106781186544,3.14018491736755E-15));
#17440=DIRECTION('center_axis',(0.,1.,0.));
#17441=DIRECTION('ref_axis',(-9.51619735392991E-16,0.,-1.));
#17442=DIRECTION('center_axis',(-0.707106781186546,0.707106781186549,0.));
#17443=DIRECTION('ref_axis',(0.,0.,1.));
#17444=DIRECTION('',(0.,0.,1.));
#17445=DIRECTION('',(0.707106781186549,0.707106781186546,0.));
#17446=DIRECTION('center_axis',(0.,-1.,0.));
#17447=DIRECTION('ref_axis',(-1.,0.,6.3441315692866E-16));
#17448=DIRECTION('',(0.,0.707106781186548,-0.707106781186548));
#17449=DIRECTION('center_axis',(0.,1.,0.));
#17450=DIRECTION('ref_axis',(-1.,0.,6.3441315692866E-16));
#17451=DIRECTION('center_axis',(0.,0.707106781186548,0.707106781186548));
#17452=DIRECTION('ref_axis',(1.,0.,0.));
#17453=DIRECTION('',(1.,0.,0.));
#17454=DIRECTION('center_axis',(0.,0.,-1.));
#17455=DIRECTION('ref_axis',(1.,0.,0.));
#17456=DIRECTION('',(0.,-1.,0.));
#17457=DIRECTION('',(0.907485212973028,0.420084025208408,0.));
#17458=DIRECTION('',(1.,0.,0.));
#17459=DIRECTION('',(0.907485212973032,-0.420084025208399,0.));
#17460=DIRECTION('',(0.,-1.,0.));
#17461=DIRECTION('center_axis',(0.,-1.,0.));
#17462=DIRECTION('ref_axis',(1.,0.,-1.26882631385732E-15));
#17463=DIRECTION('',(0.,-1.,0.));
#17464=DIRECTION('center_axis',(0.,-1.,0.));
#17465=DIRECTION('ref_axis',(1.,0.,-1.26882631385732E-15));
#17466=DIRECTION('center_axis',(1.,0.,0.));
#17467=DIRECTION('ref_axis',(0.,0.,1.));
#17468=DIRECTION('',(0.,-1.,0.));
#17469=DIRECTION('',(0.,0.42008402520841,0.907485212973027));
#17470=DIRECTION('',(0.,0.,1.));
#17471=DIRECTION('',(0.,-0.420084025208404,0.90748521297303));
#17472=DIRECTION('center_axis',(0.,-1.,0.));
#17473=DIRECTION('ref_axis',(1.26882631385732E-15,0.,1.));
#17474=DIRECTION('',(0.,-1.,0.));
#17475=DIRECTION('center_axis',(0.,-1.,0.));
#17476=DIRECTION('ref_axis',(1.26882631385732E-15,0.,1.));
#17477=DIRECTION('',(0.,0.420084025208396,-0.907485212973033));
#17478=DIRECTION('',(0.499919264427449,-0.739339319775861,0.451063298537672));
#17479=DIRECTION('center_axis',(0.,1.,0.));
#17480=DIRECTION('ref_axis',(-9.5161973539299E-16,0.,-1.));
#17481=DIRECTION('',(0.437408882639852,-0.707106781186545,0.55558389950372));
#17482=DIRECTION('center_axis',(0.,1.,0.));
#17483=DIRECTION('ref_axis',(-9.51619735392991E-16,0.,-1.));
#17484=DIRECTION('',(-0.555583899503719,0.707106781186547,-0.43740888263985));
#17485=DIRECTION('center_axis',(0.,-1.,0.));
#17486=DIRECTION('ref_axis',(-9.51619735392991E-16,0.,-1.));
#17487=DIRECTION('',(-0.451063298380524,0.739339319957295,-0.499919264300915));
#17488=DIRECTION('center_axis',(1.,0.,0.));
#17489=DIRECTION('ref_axis',(0.,-0.70710678118655,-0.707106781186545));
#17490=DIRECTION('',(-1.,0.,0.));
#17491=DIRECTION('center_axis',(0.,-1.,0.));
#17492=DIRECTION('ref_axis',(-9.51619735392991E-16,0.,-1.));
#17493=DIRECTION('',(0.,-1.,0.));
#17494=DIRECTION('',(0.,-0.420084025208414,-0.907485212973025));
#17495=DIRECTION('',(-0.907485212973031,0.420084025208401,0.));
#17496=DIRECTION('',(0.451063298380521,-0.739339319957302,-0.499919264300906));
#17497=DIRECTION('center_axis',(0.,1.,0.));
#17498=DIRECTION('ref_axis',(-1.,0.,6.3441315692866E-16));
#17499=DIRECTION('',(0.555583899503716,-0.707106781186546,-0.437408882639856));
#17500=DIRECTION('center_axis',(0.,1.,0.));
#17501=DIRECTION('ref_axis',(-1.,0.,6.3441315692866E-16));
#17502=DIRECTION('',(-0.437408882639855,0.707106781186547,0.555583899503715));
#17503=DIRECTION('center_axis',(0.,-1.,0.));
#17504=DIRECTION('ref_axis',(-1.,0.,6.3441315692866E-16));
#17505=DIRECTION('',(-0.499919264427448,0.739339319775853,0.451063298537686));
#17506=DIRECTION('center_axis',(0.,0.,-1.));
#17507=DIRECTION('ref_axis',(-0.707106781186546,-0.707106781186549,0.));
#17508=DIRECTION('',(0.,0.,1.));
#17509=DIRECTION('',(0.,0.,-1.));
#17510=DIRECTION('center_axis',(-1.,0.,0.));
#17511=DIRECTION('ref_axis',(0.,0.,-1.));
#17512=DIRECTION('',(0.,-1.,0.));
#17513=DIRECTION('center_axis',(0.,-1.,0.));
#17514=DIRECTION('ref_axis',(-1.,0.,6.3441315692866E-16));
#17515=DIRECTION('',(0.,-1.,0.));
#17516=DIRECTION('center_axis',(0.,-1.,0.));
#17517=DIRECTION('ref_axis',(1.,0.,-9.51619735392991E-16));
#17518=DIRECTION('',(0.,-0.707106781186548,-0.707106781186548));
#17519=DIRECTION('center_axis',(0.,-1.,0.));
#17520=DIRECTION('ref_axis',(1.,0.,-9.51619735392991E-16));
#17521=DIRECTION('',(-0.707106781186548,0.707106781186548,7.8504622934189E-16));
#17522=DIRECTION('center_axis',(0.,-0.707106781186549,0.707106781186546));
#17523=DIRECTION('ref_axis',(1.,0.,0.));
#17524=DIRECTION('',(7.85046229341889E-16,-0.707106781186546,-0.707106781186549));
#17525=DIRECTION('',(1.,0.,0.));
#17526=DIRECTION('center_axis',(0.,-1.,0.));
#17527=DIRECTION('ref_axis',(-3.96508223080413E-16,0.,-1.));
#17528=DIRECTION('',(-0.70710678118655,-0.707106781186545,-7.85046229341888E-16));
#17529=DIRECTION('center_axis',(0.,-1.,0.));
#17530=DIRECTION('ref_axis',(-3.96508223080413E-16,0.,-1.));
#17531=DIRECTION('center_axis',(0.707106781186547,-0.707106781186548,0.));
#17532=DIRECTION('ref_axis',(0.,0.,-1.));
#17533=DIRECTION('',(-0.707106781186548,-0.707106781186547,7.85046229341889E-16));
#17534=DIRECTION('',(0.,0.,-1.));
#17535=DIRECTION('center_axis',(0.,-1.,0.));
#17536=DIRECTION('ref_axis',(-1.,0.,3.1720657846433E-16));
#17537=DIRECTION('',(-3.92523114670943E-16,-0.707106781186544,0.707106781186551));
#17538=DIRECTION('center_axis',(0.,-1.,0.));
#17539=DIRECTION('ref_axis',(-1.,0.,3.1720657846433E-16));
#17540=DIRECTION('center_axis',(0.,1.,0.));
#17541=DIRECTION('ref_axis',(-1.,0.,3.1720657846433E-16));
#17542=DIRECTION('center_axis',(0.,-0.707106781186549,-0.707106781186546));
#17543=DIRECTION('ref_axis',(-1.,0.,0.));
#17544=DIRECTION('',(0.,-0.707106781186546,0.707106781186549));
#17545=DIRECTION('',(-1.,0.,0.));
#17546=DIRECTION('',(1.,0.,0.));
#17547=DIRECTION('center_axis',(0.,-1.,0.));
#17548=DIRECTION('ref_axis',(6.3441315692866E-16,0.,1.));
#17549=DIRECTION('',(0.707106781186551,-0.707106781186544,7.85046229341887E-16));
#17550=DIRECTION('center_axis',(0.,-1.,0.));
#17551=DIRECTION('ref_axis',(6.3441315692866E-16,0.,1.));
#17552=DIRECTION('center_axis',(0.,1.,0.));
#17553=DIRECTION('ref_axis',(6.3441315692866E-16,0.,1.));
#17554=DIRECTION('center_axis',(-0.707106781186548,-0.707106781186548,0.));
#17555=DIRECTION('ref_axis',(0.,0.,1.));
#17556=DIRECTION('',(0.,0.,1.));
#17557=DIRECTION('',(0.,0.,-1.));
#17558=DIRECTION('center_axis',(0.,1.,0.));
#17559=DIRECTION('ref_axis',(1.,0.,0.));
#17560=DIRECTION('center_axis',(0.,1.,0.));
#17561=DIRECTION('ref_axis',(1.,0.,-1.26882631385732E-15));
#17562=DIRECTION('',(0.,0.,-1.));
#17563=DIRECTION('center_axis',(0.,1.,0.));
#17564=DIRECTION('ref_axis',(1.26882631385732E-15,0.,1.));
#17565=DIRECTION('',(1.,0.,0.));
#17566=DIRECTION('',(-0.451063298380529,-0.739339319957298,0.499919264300905));
#17567=DIRECTION('center_axis',(0.,1.,0.));
#17568=DIRECTION('ref_axis',(1.,0.,-1.26882631385732E-15));
#17569=DIRECTION('',(-0.555583899503719,-0.707106781186544,0.437408882639855));
#17570=DIRECTION('',(0.437408882639851,0.707106781186548,-0.555583899503717));
#17571=DIRECTION('',(0.499919264427449,0.739339319775855,-0.451063298537682));
#17572=DIRECTION('center_axis',(0.,0.,1.));
#17573=DIRECTION('ref_axis',(0.707106781186548,-0.707106781186548,0.));
#17574=DIRECTION('',(-0.907485212973031,-0.420084025208402,0.));
#17575=DIRECTION('',(-0.49991926442746,-0.739339319775848,-0.451063298537683));
#17576=DIRECTION('center_axis',(0.,1.,0.));
#17577=DIRECTION('ref_axis',(1.26882631385732E-15,0.,1.));
#17578=DIRECTION('',(-0.437408882639856,-0.707106781186546,-0.555583899503715));
#17579=DIRECTION('',(0.555583899503722,0.707106781186548,0.437408882639845));
#17580=DIRECTION('',(0.451063298380523,0.739339319957298,0.499919264300911));
#17581=DIRECTION('center_axis',(-1.,0.,0.));
#17582=DIRECTION('ref_axis',(0.,-0.70710678118655,0.707106781186545));
#17583=DIRECTION('',(-1.,0.,0.));
#17584=DIRECTION('center_axis',(0.,0.,1.));
#17585=DIRECTION('ref_axis',(-1.,0.,0.));
#17586=DIRECTION('center_axis',(-1.,0.,0.));
#17587=DIRECTION('ref_axis',(0.,0.,-1.));
#17588=DIRECTION('',(0.,-1.,0.));
#17589=DIRECTION('center_axis',(0.,-1.,0.));
#17590=DIRECTION('ref_axis',(6.3441315692866E-16,0.,1.));
#17591=DIRECTION('',(0.,-1.,0.));
#17592=DIRECTION('center_axis',(0.,0.,-1.));
#17593=DIRECTION('ref_axis',(1.,0.,0.));
#17594=DIRECTION('',(0.,-1.,0.));
#17595=DIRECTION('center_axis',(0.,-1.,0.));
#17596=DIRECTION('ref_axis',(-1.,0.,3.1720657846433E-16));
#17597=DIRECTION('center_axis',(1.,0.,0.));
#17598=DIRECTION('ref_axis',(0.,0.,1.));
#17599=DIRECTION('',(0.,-1.,0.));
#17600=DIRECTION('',(0.,-1.,0.));
#17601=DIRECTION('center_axis',(0.,-1.,0.));
#17602=DIRECTION('ref_axis',(-6.5658350918692E-16,0.,-1.));
#17603=DIRECTION('',(0.,-1.,0.));
#17604=DIRECTION('center_axis',(0.,0.,1.));
#17605=DIRECTION('ref_axis',(-1.,0.,0.));
#17606=DIRECTION('center_axis',(0.,-1.,0.));
#17607=DIRECTION('ref_axis',(-1.,0.,5.96894099260836E-16));
#26844=CARTESIAN_POINT('',(0.,0.,0.));
#26845=CARTESIAN_POINT('Origin',(-5.05,-72.25,-2.));
#26846=CARTESIAN_POINT('',(-4.8,-72.5,-4.));
#26847=CARTESIAN_POINT('',(-5.3,-72.,-4.));
#26848=CARTESIAN_POINT('',(-4.8,-72.5,-4.));
#26849=CARTESIAN_POINT('',(-5.3,-72.,4.));
#26850=CARTESIAN_POINT('',(-5.3,-72.,-2.));
#26851=CARTESIAN_POINT('',(-4.8,-72.5,4.));
#26852=CARTESIAN_POINT('',(-5.3,-72.,4.));
#26853=CARTESIAN_POINT('',(-4.8,-72.5,-2.));
#26854=CARTESIAN_POINT('Origin',(2.2,-72.25,-4.));
#26855=CARTESIAN_POINT('',(2.2,-72.5,-11.));
#26856=CARTESIAN_POINT('',(2.2,-72.,-11.5));
#26857=CARTESIAN_POINT('',(2.2,-72.5,-11.));
#26858=CARTESIAN_POINT('Origin',(2.2,-72.,-4.));
#26859=CARTESIAN_POINT('Origin',(2.2,-72.5,-4.));
#26860=CARTESIAN_POINT('Origin',(21.7,-72.25,-11.25));
#26861=CARTESIAN_POINT('',(28.2,-72.5,-11.));
#26862=CARTESIAN_POINT('',(28.2,-72.,-11.5));
#26863=CARTESIAN_POINT('',(28.2,-72.5,-11.));
#26864=CARTESIAN_POINT('',(21.7,-72.,-11.5));
#26865=CARTESIAN_POINT('',(21.7,-72.5,-11.));
#26866=CARTESIAN_POINT('Origin',(28.2,-72.25,-3.99999999999999));
#26867=CARTESIAN_POINT('',(35.2,-72.5,-4.));
#26868=CARTESIAN_POINT('',(35.7,-72.,-4.));
#26869=CARTESIAN_POINT('',(35.2,-72.5,-4.));
#26870=CARTESIAN_POINT('Origin',(28.2,-72.,-3.99999999999999));
#26871=CARTESIAN_POINT('Origin',(28.2,-72.5,-3.99999999999999));
#26872=CARTESIAN_POINT('Origin',(35.45,-72.25,2.));
#26873=CARTESIAN_POINT('',(35.2,-72.5,4.));
#26874=CARTESIAN_POINT('',(35.7,-72.,4.));
#26875=CARTESIAN_POINT('',(35.2,-72.5,4.));
#26876=CARTESIAN_POINT('',(35.7,-72.,2.));
#26877=CARTESIAN_POINT('',(35.2,-72.5,2.));
#26878=CARTESIAN_POINT('Origin',(28.2,-72.25,3.99999999999999));
#26879=CARTESIAN_POINT('',(28.2,-72.5,11.));
#26880=CARTESIAN_POINT('',(28.2,-72.,11.5));
#26881=CARTESIAN_POINT('',(28.2,-72.5,11.));
#26882=CARTESIAN_POINT('Origin',(28.2,-72.,3.99999999999999));
#26883=CARTESIAN_POINT('Origin',(28.2,-72.5,3.99999999999999));
#26884=CARTESIAN_POINT('Origin',(8.7,-72.25,11.25));
#26885=CARTESIAN_POINT('',(2.2,-72.5,11.));
#26886=CARTESIAN_POINT('',(2.2,-72.,11.5));
#26887=CARTESIAN_POINT('',(2.2,-72.5,11.));
#26888=CARTESIAN_POINT('',(8.7,-72.,11.5));
#26889=CARTESIAN_POINT('',(8.7,-72.5,11.));
#26890=CARTESIAN_POINT('Origin',(2.2,-72.25,4.));
#26891=CARTESIAN_POINT('Origin',(2.2,-72.,4.));
#26892=CARTESIAN_POINT('Origin',(2.2,-72.5,4.));
#26893=CARTESIAN_POINT('Origin',(28.2,-72.,-3.99999999999999));
#26894=CARTESIAN_POINT('',(28.2,-73.5,-11.));
#26895=CARTESIAN_POINT('',(28.2,-72.,-11.));
#26896=CARTESIAN_POINT('',(35.2,-73.5,-4.));
#26897=CARTESIAN_POINT('Origin',(28.2,-73.5,-3.99999999999999));
#26898=CARTESIAN_POINT('',(35.2,-72.,-4.));
#26899=CARTESIAN_POINT('Origin',(28.2,-72.,-11.));
#26900=CARTESIAN_POINT('',(2.2,-73.5,-11.));
#26901=CARTESIAN_POINT('',(2.2,-72.,-11.));
#26902=CARTESIAN_POINT('',(21.7,-73.5,-11.));
#26903=CARTESIAN_POINT('Origin',(2.2,-72.,-4.));
#26904=CARTESIAN_POINT('',(-4.8,-73.5,-4.));
#26905=CARTESIAN_POINT('',(-4.8,-72.,-4.));
#26906=CARTESIAN_POINT('Origin',(2.2,-73.5,-4.));
#26907=CARTESIAN_POINT('Origin',(-4.8,-72.,-4.));
#26908=CARTESIAN_POINT('',(-4.8,-73.5,4.));
#26909=CARTESIAN_POINT('',(-4.8,-72.,4.));
#26910=CARTESIAN_POINT('',(-4.8,-73.5,-2.));
#26911=CARTESIAN_POINT('Origin',(15.2,-72.,0.));
#26912=CARTESIAN_POINT('',(37.5,-72.,-4.));
#26913=CARTESIAN_POINT('',(37.5,-72.,4.));
#26914=CARTESIAN_POINT('',(37.5,-72.,2.));
#26915=CARTESIAN_POINT('',(28.2,-72.,-13.3));
#26916=CARTESIAN_POINT('Origin',(28.2,-72.,-4.));
#26917=CARTESIAN_POINT('',(2.2,-72.,-13.3));
#26918=CARTESIAN_POINT('',(21.7,-72.,-13.3));
#26919=CARTESIAN_POINT('',(-7.1,-72.,-4.));
#26920=CARTESIAN_POINT('Origin',(2.20000000000001,-72.,-3.99999999999999));
#26921=CARTESIAN_POINT('',(-7.1,-72.,4.));
#26922=CARTESIAN_POINT('',(-7.1,-72.,-2.));
#26923=CARTESIAN_POINT('',(2.2,-72.,13.3));
#26924=CARTESIAN_POINT('Origin',(2.2,-72.,3.99999999999999));
#26925=CARTESIAN_POINT('',(28.2,-72.,13.3));
#26926=CARTESIAN_POINT('',(8.7,-72.,13.3));
#26927=CARTESIAN_POINT('Origin',(28.2,-72.,4.));
#26928=CARTESIAN_POINT('Origin',(28.2,-32.25,-4.));
#26929=CARTESIAN_POINT('',(37.5,-32.5,-4.));
#26930=CARTESIAN_POINT('',(38.,-32.,-4.));
#26931=CARTESIAN_POINT('',(37.5,-32.5,-4.));
#26932=CARTESIAN_POINT('',(28.2,-32.,-13.8));
#26933=CARTESIAN_POINT('Origin',(28.2,-32.,-4.));
#26934=CARTESIAN_POINT('',(28.2,-32.5,-13.3));
#26935=CARTESIAN_POINT('',(28.2,-32.,-13.8));
#26936=CARTESIAN_POINT('Origin',(28.2,-32.5,-4.));
#26937=CARTESIAN_POINT('Origin',(37.75,-32.25,2.));
#26938=CARTESIAN_POINT('',(37.5,-32.5,4.));
#26939=CARTESIAN_POINT('',(38.,-32.,4.));
#26940=CARTESIAN_POINT('',(37.5,-32.5,4.));
#26941=CARTESIAN_POINT('',(38.,-32.,2.));
#26942=CARTESIAN_POINT('',(37.5,-32.5,2.));
#26943=CARTESIAN_POINT('Origin',(28.2,-32.25,4.));
#26944=CARTESIAN_POINT('',(28.2,-32.5,13.3));
#26945=CARTESIAN_POINT('',(28.2,-32.,13.8));
#26946=CARTESIAN_POINT('',(28.2,-32.5,13.3));
#26947=CARTESIAN_POINT('Origin',(28.2,-32.,4.));
#26948=CARTESIAN_POINT('Origin',(28.2,-32.5,4.));
#26949=CARTESIAN_POINT('Origin',(8.7,-32.25,13.55));
#26950=CARTESIAN_POINT('',(2.2,-32.5,13.3));
#26951=CARTESIAN_POINT('',(2.2,-32.,13.8));
#26952=CARTESIAN_POINT('',(2.2,-32.5,13.3));
#26953=CARTESIAN_POINT('',(8.7,-32.,13.8));
#26954=CARTESIAN_POINT('',(8.7,-32.5,13.3));
#26955=CARTESIAN_POINT('Origin',(2.2,-32.25,3.99999999999999));
#26956=CARTESIAN_POINT('',(-7.1,-32.5,4.));
#26957=CARTESIAN_POINT('',(-7.6,-32.,4.));
#26958=CARTESIAN_POINT('',(-7.1,-32.5,4.));
#26959=CARTESIAN_POINT('Origin',(2.2,-32.,3.99999999999999));
#26960=CARTESIAN_POINT('Origin',(2.2,-32.5,3.99999999999999));
#26961=CARTESIAN_POINT('Origin',(-7.35,-32.25,-2.));
#26962=CARTESIAN_POINT('',(-7.1,-32.5,-4.));
#26963=CARTESIAN_POINT('',(-7.6,-32.,-4.));
#26964=CARTESIAN_POINT('',(-7.1,-32.5,-4.));
#26965=CARTESIAN_POINT('',(-7.6,-32.,-2.));
#26966=CARTESIAN_POINT('',(-7.1,-32.5,-2.));
#26967=CARTESIAN_POINT('Origin',(2.20000000000001,-32.25,-3.99999999999999));
#26968=CARTESIAN_POINT('',(2.2,-32.5,-13.3));
#26969=CARTESIAN_POINT('',(2.2,-32.,-13.8));
#26970=CARTESIAN_POINT('',(2.2,-32.5,-13.3));
#26971=CARTESIAN_POINT('Origin',(2.20000000000001,-32.,-3.99999999999999));
#26972=CARTESIAN_POINT('Origin',(2.20000000000001,-32.5,-3.99999999999999));
#26973=CARTESIAN_POINT('Origin',(21.7,-32.25,-13.55));
#26974=CARTESIAN_POINT('',(21.7,-32.,-13.8));
#26975=CARTESIAN_POINT('',(21.7,-32.5,-13.3));
#26976=CARTESIAN_POINT('Origin',(2.2,-32.,13.3));
#26977=CARTESIAN_POINT('',(28.2,-32.,13.3));
#26978=CARTESIAN_POINT('',(2.2,-32.,13.3));
#26979=CARTESIAN_POINT('Origin',(28.2,-32.,4.));
#26980=CARTESIAN_POINT('',(37.5,-32.,4.));
#26981=CARTESIAN_POINT('Origin',(37.5,-32.,4.));
#26982=CARTESIAN_POINT('',(37.5,-32.,-4.));
#26983=CARTESIAN_POINT('Origin',(28.2,-32.,-4.));
#26984=CARTESIAN_POINT('',(28.2,-32.,-13.3));
#26985=CARTESIAN_POINT('Origin',(15.2,-32.,0.));
#26986=CARTESIAN_POINT('',(41.7,-32.,20.));
#26987=CARTESIAN_POINT('',(35.2,-32.,26.5));
#26988=CARTESIAN_POINT('Origin',(35.2,-32.,20.));
#26989=CARTESIAN_POINT('',(41.7,-32.,-20.));
#26990=CARTESIAN_POINT('',(41.7,-32.,-10.));
#26991=CARTESIAN_POINT('',(35.2,-32.,-26.5));
#26992=CARTESIAN_POINT('Origin',(35.2,-32.,-20.));
#26993=CARTESIAN_POINT('',(-4.8,-32.,-26.5));
#26994=CARTESIAN_POINT('',(5.2,-32.,-26.5));
#26995=CARTESIAN_POINT('',(-11.3,-32.,-20.));
#26996=CARTESIAN_POINT('Origin',(-4.79999999999999,-32.,-20.));
#26997=CARTESIAN_POINT('',(-11.3,-32.,20.));
#26998=CARTESIAN_POINT('',(-11.3,-32.,10.));
#26999=CARTESIAN_POINT('',(-4.8,-32.,26.5));
#27000=CARTESIAN_POINT('Origin',(-4.79999999999999,-32.,20.));
#27001=CARTESIAN_POINT('',(25.2,-32.,26.5));
#27002=CARTESIAN_POINT('Origin',(35.2,-32.25,20.));
#27003=CARTESIAN_POINT('',(42.2,-32.5,20.));
#27004=CARTESIAN_POINT('',(42.2,-32.5,20.));
#27005=CARTESIAN_POINT('',(35.2,-32.5,27.));
#27006=CARTESIAN_POINT('',(35.2,-32.,26.5));
#27007=CARTESIAN_POINT('Origin',(35.2,-32.5,20.));
#27008=CARTESIAN_POINT('Origin',(41.95,-32.25,-10.));
#27009=CARTESIAN_POINT('',(42.2,-32.5,-20.));
#27010=CARTESIAN_POINT('',(42.2,-32.5,-10.));
#27011=CARTESIAN_POINT('',(42.2,-32.5,-20.));
#27012=CARTESIAN_POINT('Origin',(35.2,-32.25,-20.));
#27013=CARTESIAN_POINT('',(35.2,-32.5,-27.));
#27014=CARTESIAN_POINT('',(35.2,-32.5,-27.));
#27015=CARTESIAN_POINT('Origin',(35.2,-32.5,-20.));
#27016=CARTESIAN_POINT('Origin',(5.2,-32.25,-26.75));
#27017=CARTESIAN_POINT('',(-4.8,-32.5,-27.));
#27018=CARTESIAN_POINT('',(5.2,-32.5,-27.));
#27019=CARTESIAN_POINT('',(-4.8,-32.5,-27.));
#27020=CARTESIAN_POINT('Origin',(-4.79999999999999,-32.25,-20.));
#27021=CARTESIAN_POINT('',(-11.8,-32.5,-20.));
#27022=CARTESIAN_POINT('',(-11.8,-32.5,-20.));
#27023=CARTESIAN_POINT('Origin',(-4.79999999999999,-32.5,-20.));
#27024=CARTESIAN_POINT('Origin',(-11.55,-32.25,10.));
#27025=CARTESIAN_POINT('',(-11.8,-32.5,20.));
#27026=CARTESIAN_POINT('',(-11.8,-32.5,10.));
#27027=CARTESIAN_POINT('',(-11.8,-32.5,20.));
#27028=CARTESIAN_POINT('Origin',(-4.79999999999999,-32.25,20.));
#27029=CARTESIAN_POINT('',(-4.8,-32.5,27.));
#27030=CARTESIAN_POINT('',(-4.8,-32.5,27.));
#27031=CARTESIAN_POINT('Origin',(-4.79999999999999,-32.5,20.));
#27032=CARTESIAN_POINT('Origin',(25.2,-32.25,26.75));
#27033=CARTESIAN_POINT('',(25.2,-32.5,27.));
#27034=CARTESIAN_POINT('Origin',(-4.8,-32.,-27.));
#27035=CARTESIAN_POINT('',(35.2,-71.9490268349807,-27.));
#27036=CARTESIAN_POINT('',(35.2,-32.,-27.));
#27037=CARTESIAN_POINT('',(34.0097619285762,-72.5,-27.));
#27038=CARTESIAN_POINT('',(34.6048809642881,-72.2245134174903,-27.));
#27039=CARTESIAN_POINT('',(-3.60976192857618,-72.5,-27.));
#27040=CARTESIAN_POINT('',(5.2,-72.5,-27.));
#27041=CARTESIAN_POINT('',(-4.8,-71.9490268349807,-27.));
#27042=CARTESIAN_POINT('',(-4.20488096428809,-72.2245134174903,-27.));
#27043=CARTESIAN_POINT('',(-4.8,-32.,-27.));
#27044=CARTESIAN_POINT('Origin',(35.2,-32.,-20.));
#27045=CARTESIAN_POINT('',(42.2,-71.9490268349807,-20.));
#27046=CARTESIAN_POINT('',(42.2,-32.,-20.));
#27047=CARTESIAN_POINT('',(42.1968209160836,-72.0466857368163,-20.2109432820811));
#27048=CARTESIAN_POINT('Ctrl Pts',(42.1968209160836,-72.0466857368163,-20.2109432820811));
#27049=CARTESIAN_POINT('Ctrl Pts',(42.1968440264343,-72.0463307309993,-20.2101767301278));
#27050=CARTESIAN_POINT('Ctrl Pts',(42.196867151744,-72.0459737810207,-20.2094059772172));
#27051=CARTESIAN_POINT('Ctrl Pts',(42.1968938349779,-72.0455591055399,-20.2085105801841));
#27052=CARTESIAN_POINT('Ctrl Pts',(42.1969215748069,-72.0451280098565,-20.2075797274724));
#27053=CARTESIAN_POINT('Ctrl Pts',(42.1969531556842,-72.0446346198902,-20.2065143654833));
#27054=CARTESIAN_POINT('Ctrl Pts',(42.1969907706432,-72.0440407131694,-20.2052319554396));
#27055=CARTESIAN_POINT('Ctrl Pts',(42.1970302352795,-72.0434176016909,-20.2038864841889));
#27056=CARTESIAN_POINT('Ctrl Pts',(42.1970763351041,-72.0426839627648,-20.2023023485086));
#27057=CARTESIAN_POINT('Ctrl Pts',(42.1971297471362,-72.0418204588819,-20.2004377752349));
#27058=CARTESIAN_POINT('Ctrl Pts',(42.1971866204212,-72.0409009974715,-20.1984523722667));
#27059=CARTESIAN_POINT('Ctrl Pts',(42.1972517663276,-72.039834454825,-20.1961493535318));
#27060=CARTESIAN_POINT('Ctrl Pts',(42.1973241283667,-72.0386228526127,-20.1935330529333));
#27061=CARTESIAN_POINT('Ctrl Pts',(42.1974033531205,-72.0372963437394,-20.1906686260413));
#27062=CARTESIAN_POINT('Ctrl Pts',(42.1974911870066,-72.0357962057728,-20.1874292153276));
#27063=CARTESIAN_POINT('Ctrl Pts',(42.197584514987,-72.0341515121676,-20.1838775560355));
#27064=CARTESIAN_POINT('Ctrl Pts',(42.1976993757062,-72.0321273529655,-20.1795064538336));
#27065=CARTESIAN_POINT('Ctrl Pts',(42.197822445902,-72.0298846925147,-20.1746633732515));
#27066=CARTESIAN_POINT('Ctrl Pts',(42.1979466024095,-72.027511696443,-20.1695386381502));
#27067=CARTESIAN_POINT('Ctrl Pts',(42.1980821533145,-72.024920919917,-20.1639435832062));
#27068=CARTESIAN_POINT('Ctrl Pts',(42.1982187728114,-72.0221774130799,-20.1580184730275));
#27069=CARTESIAN_POINT('Ctrl Pts',(42.1983487795842,-72.0194065699845,-20.1520340727998));
#27070=CARTESIAN_POINT('Ctrl Pts',(42.1984473485597,-72.0173057627784,-20.1474967999592));
#27071=CARTESIAN_POINT('Ctrl Pts',(42.198542156045,-72.0151898308564,-20.1429267194319));
#27072=CARTESIAN_POINT('Ctrl Pts',(42.198631372502,-72.0131013188952,-20.1384157210408));
#27073=CARTESIAN_POINT('Ctrl Pts',(42.1987118838834,-72.0112165883326,-20.1343448721814));
#27074=CARTESIAN_POINT('Ctrl Pts',(42.1987878612489,-72.0093544513594,-20.1303227080405));
#27075=CARTESIAN_POINT('Ctrl Pts',(42.198859022311,-72.0075300311515,-20.1263819046223));
#27076=CARTESIAN_POINT('Ctrl Pts',(42.1989256149734,-72.0058227351212,-20.1226940930081));
#27077=CARTESIAN_POINT('Ctrl Pts',(42.1989880057221,-72.0041486403603,-20.1190779023671));
#27078=CARTESIAN_POINT('Ctrl Pts',(42.1990467044472,-72.0025022857799,-20.1155215519585));
#27079=CARTESIAN_POINT('Ctrl Pts',(42.1991060919784,-72.0008366118852,-20.1119234691961));
#27080=CARTESIAN_POINT('Ctrl Pts',(42.199161711364,-71.999199728262,-20.1083874932512));
#27081=CARTESIAN_POINT('Ctrl Pts',(42.1992146913247,-71.9975625728967,-20.1048508690683));
#27082=CARTESIAN_POINT('Ctrl Pts',(42.1992663579433,-71.9959660016516,-20.1014019157222));
#27083=CARTESIAN_POINT('Ctrl Pts',(42.19931563984,-71.9943651666196,-20.0979436948257));
#27084=CARTESIAN_POINT('Ctrl Pts',(42.1993631272831,-71.9927356970358,-20.0944235798369));
#27085=CARTESIAN_POINT('Ctrl Pts',(42.1994134018495,-71.9910105909616,-20.0906968629903));
#27086=CARTESIAN_POINT('Ctrl Pts',(42.1994616361791,-71.9892535447084,-20.0869011062894));
#27087=CARTESIAN_POINT('Ctrl Pts',(42.1995075723881,-71.9874609701946,-20.0830285738872));
#27088=CARTESIAN_POINT('Ctrl Pts',(42.1995572904834,-71.985520814653,-20.078837219418));
#27089=CARTESIAN_POINT('Ctrl Pts',(42.1996042772797,-71.9835392694509,-20.0745564223781));
#27090=CARTESIAN_POINT('Ctrl Pts',(42.1996476627856,-71.9815377443591,-20.0702324487676));
#27091=CARTESIAN_POINT('Ctrl Pts',(42.1996984016497,-71.9791969831448,-20.0651756099797));
#27092=CARTESIAN_POINT('Ctrl Pts',(42.1997441440131,-71.976829265232,-20.0600605172026));
#27093=CARTESIAN_POINT('Ctrl Pts',(42.1997837204606,-71.9744988699025,-20.0550260554195));
#27094=CARTESIAN_POINT('Ctrl Pts',(42.1998416179811,-71.9710896677196,-20.0476609968461));
#27095=CARTESIAN_POINT('Ctrl Pts',(42.1998859839155,-71.9677638296965,-20.0404760377688));
#27096=CARTESIAN_POINT('Ctrl Pts',(42.199917487043,-71.9647604963968,-20.033987859449));
#27097=CARTESIAN_POINT('Ctrl Pts',(42.1999376069614,-71.962842375057,-20.0298440924906));
#27098=CARTESIAN_POINT('Ctrl Pts',(42.1999526242593,-71.9610565580335,-20.0259861725222));
#27099=CARTESIAN_POINT('Ctrl Pts',(42.1999637788496,-71.9594514906783,-20.022518765367));
#27100=CARTESIAN_POINT('Ctrl Pts',(42.1999740893287,-71.9579678850109,-20.0193137503938));
#27101=CARTESIAN_POINT('Ctrl Pts',(42.1999811326703,-71.9566391654817,-20.0164433694763));
#27102=CARTESIAN_POINT('Ctrl Pts',(42.1999861098761,-71.9554826093195,-20.0139449468308));
#27103=CARTESIAN_POINT('Ctrl Pts',(42.1999904546681,-71.9544730074947,-20.0117639787599));
#27104=CARTESIAN_POINT('Ctrl Pts',(42.1999932364772,-71.9535945583467,-20.00986636539));
#27105=CARTESIAN_POINT('Ctrl Pts',(42.1999951540824,-71.9528401206128,-20.0082366754871));
#27106=CARTESIAN_POINT('Ctrl Pts',(42.1999969972036,-71.952114986876,-20.0066702862729));
#27107=CARTESIAN_POINT('Ctrl Pts',(42.1999980448829,-71.9515045768435,-20.0053517545771));
#27108=CARTESIAN_POINT('Ctrl Pts',(42.1999987249728,-71.9509829203972,-20.0042249709246));
#27109=CARTESIAN_POINT('Ctrl Pts',(42.1999993730205,-71.9504858415435,-20.0031512751422));
#27110=CARTESIAN_POINT('Ctrl Pts',(42.1999996854038,-71.9500694193736,-20.0022518343658));
#27111=CARTESIAN_POINT('Ctrl Pts',(42.1999998528112,-71.9496914618382,-20.001435493955));
#27112=CARTESIAN_POINT('Ctrl Pts',(42.1999999551045,-71.9494605131145,-20.0009366739598));
#27113=CARTESIAN_POINT('Ctrl Pts',(42.2,-71.9492435363225,-20.0004680394446));
#27114=CARTESIAN_POINT('Ctrl Pts',(42.2,-71.9490268349807,-20.));
#27115=CARTESIAN_POINT('',(41.0736851473658,-73.4473505177094,-23.8078632839972));
#27116=CARTESIAN_POINT('Ctrl Pts',(41.0736851473658,-73.4473505177094,-23.8078632839972));
#27117=CARTESIAN_POINT('Ctrl Pts',(41.4091108998595,-73.3524777845863,-23.2904641250657));
#27118=CARTESIAN_POINT('Ctrl Pts',(41.9708821659981,-72.9316902782726,-22.1114790525524));
#27119=CARTESIAN_POINT('Ctrl Pts',(42.1783555363975,-72.3303386029005,-20.8234252418586));
#27120=CARTESIAN_POINT('Ctrl Pts',(42.1968209160836,-72.0466857368163,-20.2109432820811));
#27121=CARTESIAN_POINT('',(40.7,-73.5,-24.3301270189222));
#27122=CARTESIAN_POINT('Ctrl Pts',(40.7,-73.5,-24.3301270189222));
#27123=CARTESIAN_POINT('Ctrl Pts',(40.8292080416589,-73.5,-24.1660107641291));
#27124=CARTESIAN_POINT('Ctrl Pts',(40.9547480121633,-73.4809910208687,-23.9913255651788));
#27125=CARTESIAN_POINT('Ctrl Pts',(41.0736851473658,-73.4473505177094,-23.8078632839972));
#27126=CARTESIAN_POINT('',(39.5301270189222,-73.5,-25.5));
#27127=CARTESIAN_POINT('Origin',(35.2,-73.5,-20.));
#27128=CARTESIAN_POINT('',(39.0078632855922,-73.4473505180018,-25.8736851463318));
#27129=CARTESIAN_POINT('Ctrl Pts',(39.0078632855922,-73.4473505180018,-25.8736851463318));
#27130=CARTESIAN_POINT('Ctrl Pts',(39.195551811226,-73.4817659650606,-25.7520081704499));
#27131=CARTESIAN_POINT('Ctrl Pts',(39.3719134220716,-73.5,-25.6245609037243));
#27132=CARTESIAN_POINT('Ctrl Pts',(39.5301270189222,-73.5,-25.5));
#27133=CARTESIAN_POINT('',(35.4109442661894,-72.0466861925664,-26.9968208864142));
#27134=CARTESIAN_POINT('Ctrl Pts',(35.4109442661894,-72.0466861925664,-26.9968208864142));
#27135=CARTESIAN_POINT('Ctrl Pts',(35.7966135491349,-72.2252974952159,-26.9851935023203));
#27136=CARTESIAN_POINT('Ctrl Pts',(36.2129500341219,-72.4189119678641,-26.93930292622));
#27137=CARTESIAN_POINT('Ctrl Pts',(37.155472782663,-72.8367867066598,-26.7392783613268));
#27138=CARTESIAN_POINT('Ctrl Pts',(37.926965678302,-73.1628447118167,-26.4889617424396));
#27139=CARTESIAN_POINT('Ctrl Pts',(38.7159981118503,-73.3938327528572,-26.0628990132224));
#27140=CARTESIAN_POINT('Ctrl Pts',(39.0078632855927,-73.4473505180019,-25.8736851463315));
#27141=CARTESIAN_POINT('Ctrl Pts',(35.2,-71.9490268349807,-27.));
#27142=CARTESIAN_POINT('Ctrl Pts',(35.2007669707035,-71.9493819403517,-27.));
#27143=CARTESIAN_POINT('Ctrl Pts',(35.2015381410139,-71.9497389896615,-26.9999998883361));
#27144=CARTESIAN_POINT('Ctrl Pts',(35.2024340110129,-71.9501537584991,-26.9999995768279));
#27145=CARTESIAN_POINT('Ctrl Pts',(35.2033653543852,-71.9505849507574,-26.999999252985));
#27146=CARTESIAN_POINT('Ctrl Pts',(35.2044312667571,-71.9510784307137,-26.999998715007));
#27147=CARTESIAN_POINT('Ctrl Pts',(35.2057143192196,-71.9516724170336,-26.9999976676107));
#27148=CARTESIAN_POINT('Ctrl Pts',(35.2070604622019,-71.9522956109712,-26.9999965687117));
#27149=CARTESIAN_POINT('Ctrl Pts',(35.2086453700289,-71.9530293205579,-26.9999949098187));
#27150=CARTESIAN_POINT('Ctrl Pts',(35.2105108197961,-71.953892881673,-26.9999921087575));
#27151=CARTESIAN_POINT('Ctrl Pts',(35.2124971503262,-71.9548124013714,-26.9999891261881));
#27152=CARTESIAN_POINT('Ctrl Pts',(35.2148012127258,-71.9558789862511,-26.9999848410617));
#27153=CARTESIAN_POINT('Ctrl Pts',(35.2174186444992,-71.9570906156705,-26.9999783278824));
#27154=CARTESIAN_POINT('Ctrl Pts',(35.2202842926812,-71.9584171463859,-26.9999711970451));
#27155=CARTESIAN_POINT('Ctrl Pts',(35.2235250241412,-71.9599172861367,-26.9999613711321));
#27156=CARTESIAN_POINT('Ctrl Pts',(35.2270780387911,-71.9615619664984,-26.9999476269337));
#27157=CARTESIAN_POINT('Ctrl Pts',(35.2314506214448,-71.9635860225548,-26.9999307123839));
#27158=CARTESIAN_POINT('Ctrl Pts',(35.2362951915127,-71.9658285383685,-26.9999077806186));
#27159=CARTESIAN_POINT('Ctrl Pts',(35.2414213179411,-71.968201373194,-26.9998774471001));
#27160=CARTESIAN_POINT('Ctrl Pts',(35.2470187031861,-71.9707923492119,-26.9998443249382));
#27161=CARTESIAN_POINT('Ctrl Pts',(35.2529461190972,-71.9735360807742,-26.9998023221268));
#27162=CARTESIAN_POINT('Ctrl Pts',(35.2589325903827,-71.9763071508733,-26.9997519205891));
#27163=CARTESIAN_POINT('Ctrl Pts',(35.2634711104776,-71.9784079806826,-26.9997137096998));
#27164=CARTESIAN_POINT('Ctrl Pts',(35.2680423000474,-71.9805239342997,-26.9996707497673));
#27165=CARTESIAN_POINT('Ctrl Pts',(35.2725542349323,-71.9826124675568,-26.9996239815431));
#27166=CARTESIAN_POINT('Ctrl Pts',(35.2766259050606,-71.984497206298,-26.9995817768601));
#27167=CARTESIAN_POINT('Ctrl Pts',(35.2806487513006,-71.9863593514082,-26.9995365071789));
#27168=CARTESIAN_POINT('Ctrl Pts',(35.2845900895339,-71.9881837792468,-26.9994888753932));
#27169=CARTESIAN_POINT('Ctrl Pts',(35.2882783929648,-71.9898910784073,-26.9994443015788));
#27170=CARTESIAN_POINT('Ctrl Pts',(35.2918949473981,-71.9915651760262,-26.9993976862506));
#27171=CARTESIAN_POINT('Ctrl Pts',(35.2954515321382,-71.993211531325,-26.9993491843894));
#27172=CARTESIAN_POINT('Ctrl Pts',(35.2990489039404,-71.994876767095,-26.9993001263068));
#27173=CARTESIAN_POINT('Ctrl Pts',(35.3025840722509,-71.9965132267008,-26.9992491748665));
#27174=CARTESIAN_POINT('Ctrl Pts',(35.3061197298406,-71.9981499419665,-26.9991955682734));
#27175=CARTESIAN_POINT('Ctrl Pts',(35.3095686516303,-71.999746505774,-26.9991432767429));
#27176=CARTESIAN_POINT('Ctrl Pts',(35.313026689874,-72.0013473181754,-26.9990883234737));
#27177=CARTESIAN_POINT('Ctrl Pts',(35.3165464873944,-72.0029767588717,-26.999029712487));
#27178=CARTESIAN_POINT('Ctrl Pts',(35.3202728437031,-72.0047018230503,-26.9989676619234));
#27179=CARTESIAN_POINT('Ctrl Pts',(35.3240680871851,-72.006458819974,-26.9989014928217));
#27180=CARTESIAN_POINT('Ctrl Pts',(35.3279399692184,-72.0082513459315,-26.9988307140748));
#27181=CARTESIAN_POINT('Ctrl Pts',(35.3321305670788,-72.010191424523,-26.9987541091413));
#27182=CARTESIAN_POINT('Ctrl Pts',(35.3364104437453,-72.0121728926466,-26.9986720801898));
#27183=CARTESIAN_POINT('Ctrl Pts',(35.3407333634553,-72.0141743492423,-26.9985851513296));
#27184=CARTESIAN_POINT('Ctrl Pts',(35.3457888070745,-72.0165149550492,-26.9984834922701));
#27185=CARTESIAN_POINT('Ctrl Pts',(35.3509023169183,-72.0188825276478,-26.9983750851363));
#27186=CARTESIAN_POINT('Ctrl Pts',(35.3559351026816,-72.0212128042074,-26.9982629447422));
#27187=CARTESIAN_POINT('Ctrl Pts',(35.3632986629101,-72.0246222741515,-26.9980988700955));
#27188=CARTESIAN_POINT('Ctrl Pts',(35.3704818772113,-72.0279484172625,-26.9979266950892));
#27189=CARTESIAN_POINT('Ctrl Pts',(35.3769682776864,-72.0309520300502,-26.9977626587855));
#27190=CARTESIAN_POINT('Ctrl Pts',(35.3811109071277,-72.0328703289298,-26.9976578947298));
#27191=CARTESIAN_POINT('Ctrl Pts',(35.3849676793297,-72.0346563122552,-26.9975566436896));
#27192=CARTESIAN_POINT('Ctrl Pts',(35.3884339927027,-72.0362615170312,-26.9974632996818));
#27193=CARTESIAN_POINT('Ctrl Pts',(35.3916379986998,-72.0377452506627,-26.9973770193232));
#27194=CARTESIAN_POINT('Ctrl Pts',(35.3945074173725,-72.0390740730493,-26.9972975574334));
#27195=CARTESIAN_POINT('Ctrl Pts',(35.3970049626025,-72.0402306971659,-26.9972272397508));
#27196=CARTESIAN_POINT('Ctrl Pts',(35.3991850734024,-72.0412403160099,-26.9971658593451));
#27197=CARTESIAN_POINT('Ctrl Pts',(35.4010819183648,-72.0421187666732,-26.9971114553097));
#27198=CARTESIAN_POINT('Ctrl Pts',(35.4027109342665,-72.0428731874732,-26.9970642613262));
#27199=CARTESIAN_POINT('Ctrl Pts',(35.404276671081,-72.0435983028137,-26.997018900592));
#27200=CARTESIAN_POINT('Ctrl Pts',(35.4055946392623,-72.0442086780501,-26.9969802139163));
#27201=CARTESIAN_POINT('Ctrl Pts',(35.4067209262391,-72.0447302826942,-26.9969469383907));
#27202=CARTESIAN_POINT('Ctrl Pts',(35.4077941440434,-72.0452273100082,-26.9969152307644));
#27203=CARTESIAN_POINT('Ctrl Pts',(35.40869316907,-72.0456436658995,-26.9968884389805));
#27204=CARTESIAN_POINT('Ctrl Pts',(35.4095091096287,-72.0460215435592,-26.9968640070379));
#27205=CARTESIAN_POINT('Ctrl Pts',(35.4100078256831,-72.0462525084911,-26.9968490738398));
#27206=CARTESIAN_POINT('Ctrl Pts',(35.4104763443426,-72.0464694884255,-26.9968349935969));
#27207=CARTESIAN_POINT('Ctrl Pts',(35.4109442661894,-72.0466861925664,-26.9968208864142));
#27208=CARTESIAN_POINT('Origin',(42.2,-32.,-20.));
#27209=CARTESIAN_POINT('',(42.2,-71.9490268349807,20.));
#27210=CARTESIAN_POINT('',(42.2,-32.,20.));
#27211=CARTESIAN_POINT('',(42.2,-72.5,18.8097619285762));
#27212=CARTESIAN_POINT('',(42.2,-72.2245134174903,19.4048809642881));
#27213=CARTESIAN_POINT('',(42.2,-72.5,-18.8097619285762));
#27214=CARTESIAN_POINT('',(42.2,-72.5,-10.));
#27215=CARTESIAN_POINT('',(42.2,-72.2245134174903,-19.4048809642881));
#27216=CARTESIAN_POINT('Origin',(35.2,-32.,20.));
#27217=CARTESIAN_POINT('',(35.2,-71.9490268349807,27.));
#27218=CARTESIAN_POINT('',(35.2,-32.,27.));
#27219=CARTESIAN_POINT('',(35.4109431177646,-72.046685660721,26.9968209210375));
#27220=CARTESIAN_POINT('Ctrl Pts',(35.4109431177646,-72.046685660721,26.9968209210375));
#27221=CARTESIAN_POINT('Ctrl Pts',(35.4101765648703,-72.0463306544709,26.9968440313985));
#27222=CARTESIAN_POINT('Ctrl Pts',(35.4094058110184,-72.0459737040598,26.9968671567182));
#27223=CARTESIAN_POINT('Ctrl Pts',(35.4085104131101,-72.0455590281861,26.9968938399567));
#27224=CARTESIAN_POINT('Ctrl Pts',(35.407579559468,-72.0451279320849,26.9969215797913));
#27225=CARTESIAN_POINT('Ctrl Pts',(35.406514196614,-72.0446345417411,26.9969531606685));
#27226=CARTESIAN_POINT('Ctrl Pts',(35.4052317858403,-72.0440406347175,26.9969907756178));
#27227=CARTESIAN_POINT('Ctrl Pts',(35.4038863137786,-72.0434175229004,26.9970302402452));
#27228=CARTESIAN_POINT('Ctrl Pts',(35.4023021774198,-72.0426838837104,26.9970763400508));
#27229=CARTESIAN_POINT('Ctrl Pts',(35.4004376036754,-72.0418203796692,26.9971297520507));
#27230=CARTESIAN_POINT('Ctrl Pts',(35.398452200092,-72.0409009180375,26.9971866253045));
#27231=CARTESIAN_POINT('Ctrl Pts',(35.3961491809414,-72.0398343752723,26.9972517711657));
#27232=CARTESIAN_POINT('Ctrl Pts',(35.3935328802145,-72.0386227730735,26.9973241331437));
#27233=CARTESIAN_POINT('Ctrl Pts',(35.3906684528407,-72.0372962640568,26.9974033578401));
#27234=CARTESIAN_POINT('Ctrl Pts',(35.3874290419011,-72.0357961260639,26.9974911916518));
#27235=CARTESIAN_POINT('Ctrl Pts',(35.3838773827663,-72.0341514325885,26.9975845195401));
#27236=CARTESIAN_POINT('Ctrl Pts',(35.379506277065,-72.0321272718359,26.9976993802429));
#27237=CARTESIAN_POINT('Ctrl Pts',(35.3746631927677,-72.0298846097018,26.9978224504091));
#27238=CARTESIAN_POINT('Ctrl Pts',(35.3695384544159,-72.02751161209,26.9979466068608));
#27239=CARTESIAN_POINT('Ctrl Pts',(35.3639434120815,-72.0249208413645,26.9980821573134));
#27240=CARTESIAN_POINT('Ctrl Pts',(35.3580183169952,-72.0221773413901,26.998218776321));
#27241=CARTESIAN_POINT('Ctrl Pts',(35.3520339326916,-72.0194065054176,26.998348782628));
#27242=CARTESIAN_POINT('Ctrl Pts',(35.3474966654497,-72.0173057006142,26.998447351391));
#27243=CARTESIAN_POINT('Ctrl Pts',(35.3429265908979,-72.0151897711979,26.998542158666));
#27244=CARTESIAN_POINT('Ctrl Pts',(35.3384155986028,-72.0131012617228,26.9986313749235));
#27245=CARTESIAN_POINT('Ctrl Pts',(35.3343447547669,-72.0112165331826,26.9987118861344));
#27246=CARTESIAN_POINT('Ctrl Pts',(35.3303225957582,-72.0093543982207,26.9987878633368));
#27247=CARTESIAN_POINT('Ctrl Pts',(35.326381797399,-72.0075299799367,26.9988590242472));
#27248=CARTESIAN_POINT('Ctrl Pts',(35.3226939903455,-72.0058226856266,26.9989256167707));
#27249=CARTESIAN_POINT('Ctrl Pts',(35.3190778042077,-72.0041485925122,26.99898800739));
#27250=CARTESIAN_POINT('Ctrl Pts',(35.3155214580876,-72.0025022394492,26.9990467059966));
#27251=CARTESIAN_POINT('Ctrl Pts',(35.3119233667752,-72.0008365611229,26.9991060936207));
#27252=CARTESIAN_POINT('Ctrl Pts',(35.3083873825375,-71.9991996731568,26.9991617130831));
#27253=CARTESIAN_POINT('Ctrl Pts',(35.3048507493789,-71.9975625131321,26.9992146931177));
#27254=CARTESIAN_POINT('Ctrl Pts',(35.3014017990027,-71.9959659427698,26.9992663596328));
#27255=CARTESIAN_POINT('Ctrl Pts',(35.2979435804289,-71.9943651083224,26.9993156414398));
#27256=CARTESIAN_POINT('Ctrl Pts',(35.2944234673532,-71.9927356391638,26.9993631288006));
#27257=CARTESIAN_POINT('Ctrl Pts',(35.2906967521995,-71.9910105333859,26.9994134032842));
#27258=CARTESIAN_POINT('Ctrl Pts',(35.2869009967207,-71.9892534872448,26.9994616375389));
#27259=CARTESIAN_POINT('Ctrl Pts',(35.2830284653437,-71.9874609128098,26.9995075736756));
#27260=CARTESIAN_POINT('Ctrl Pts',(35.2788371112672,-71.9855207570216,26.9995572917012));
#27261=CARTESIAN_POINT('Ctrl Pts',(35.2745563143599,-71.9835392115203,26.9996042784301));
#27262=CARTESIAN_POINT('Ctrl Pts',(35.2702323409792,-71.9815376862603,26.9996476638671));
#27263=CARTESIAN_POINT('Ctrl Pts',(35.2651754999054,-71.9791969236667,26.9996984026762));
#27264=CARTESIAN_POINT('Ctrl Pts',(35.2600604049209,-71.9768292045288,26.9997441449775));
#27265=CARTESIAN_POINT('Ctrl Pts',(35.2550259417389,-71.9744988084769,26.9997837213542));
#27266=CARTESIAN_POINT('Ctrl Pts',(35.2476608969128,-71.9710896125479,26.999841618647));
#27267=CARTESIAN_POINT('Ctrl Pts',(35.2404759526217,-71.9677637815365,26.9998859843948));
#27268=CARTESIAN_POINT('Ctrl Pts',(35.2339877884408,-71.9647604551991,26.9999174873878));
#27269=CARTESIAN_POINT('Ctrl Pts',(35.2298440288371,-71.9628423375302,26.9999376072285));
#27270=CARTESIAN_POINT('Ctrl Pts',(35.225986116163,-71.9610565242505,26.9999526244651));
#27271=CARTESIAN_POINT('Ctrl Pts',(35.2225187158526,-71.9594514605142,26.9999637790089));
#27272=CARTESIAN_POINT('Ctrl Pts',(35.2193137088523,-71.9579678589538,26.9999740894397));
#27273=CARTESIAN_POINT('Ctrl Pts',(35.2164433351698,-71.9566391432609,26.9999811327487));
#27274=CARTESIAN_POINT('Ctrl Pts',(35.2139449186996,-71.9554825904979,26.9999861099321));
#27275=CARTESIAN_POINT('Ctrl Pts',(35.211763953714,-71.9544729905733,26.9999904547092));
#27276=CARTESIAN_POINT('Ctrl Pts',(35.209866343227,-71.9535945432724,26.9999932365079));
#27277=CARTESIAN_POINT('Ctrl Pts',(35.2082366558696,-71.9528401072575,26.9999951541055));
#27278=CARTESIAN_POINT('Ctrl Pts',(35.2066702690583,-71.9521149751525,26.9999969972195));
#27279=CARTESIAN_POINT('Ctrl Pts',(35.2053517394672,-71.9515045666398,26.9999980448942));
#27280=CARTESIAN_POINT('Ctrl Pts',(35.2042249574883,-71.9509829115285,26.9999987249809));
#27281=CARTESIAN_POINT('Ctrl Pts',(35.2031512632312,-71.9504858339147,26.9999993730257));
#27282=CARTESIAN_POINT('Ctrl Pts',(35.2022518236115,-71.9500694128274,26.9999996854072));
#27283=CARTESIAN_POINT('Ctrl Pts',(35.2014354838484,-71.9496914561438,26.9999998528133));
#27284=CARTESIAN_POINT('Ctrl Pts',(35.2009366676327,-71.9494605095072,26.9999999551051));
#27285=CARTESIAN_POINT('Ctrl Pts',(35.2004680362892,-71.9492435345226,27.));
#27286=CARTESIAN_POINT('Ctrl Pts',(35.2,-71.9490268349807,27.));
#27287=CARTESIAN_POINT('',(39.0078632855922,-73.4473505180018,25.8736851463318));
#27288=CARTESIAN_POINT('Ctrl Pts',(39.0078632855927,-73.4473505180019,25.8736851463315));
#27289=CARTESIAN_POINT('Ctrl Pts',(38.7006130536539,-73.3910116765338,26.0728730238806));
#27290=CARTESIAN_POINT('Ctrl Pts',(38.1887966829792,-73.2378094420153,26.3429260072132));
#27291=CARTESIAN_POINT('Ctrl Pts',(37.0808170189174,-72.8203441337222,26.7897806502721));
#27292=CARTESIAN_POINT('Ctrl Pts',(36.0964746307403,-72.3641692597616,26.9761532269083));
#27293=CARTESIAN_POINT('Ctrl Pts',(35.4109431177646,-72.046685660721,26.9968209210375));
#27294=CARTESIAN_POINT('',(39.5301270189222,-73.5,25.5));
#27295=CARTESIAN_POINT('Ctrl Pts',(39.5301270189222,-73.5,25.5));
#27296=CARTESIAN_POINT('Ctrl Pts',(39.3719134220716,-73.5,25.6245609037243));
#27297=CARTESIAN_POINT('Ctrl Pts',(39.195551811226,-73.4817659650606,25.75200817045));
#27298=CARTESIAN_POINT('Ctrl Pts',(39.0078632855922,-73.4473505180018,25.8736851463318));
#27299=CARTESIAN_POINT('',(40.7,-73.5,24.3301270189222));
#27300=CARTESIAN_POINT('Origin',(35.2,-73.5,20.));
#27301=CARTESIAN_POINT('',(41.0736851473658,-73.4473505177094,23.8078632839972));
#27302=CARTESIAN_POINT('Ctrl Pts',(41.0736851473658,-73.4473505177094,23.8078632839972));
#27303=CARTESIAN_POINT('Ctrl Pts',(40.9547480121633,-73.4809910208687,23.9913255651787));
#27304=CARTESIAN_POINT('Ctrl Pts',(40.8292080416589,-73.5,24.1660107641291));
#27305=CARTESIAN_POINT('Ctrl Pts',(40.7,-73.5,24.3301270189222));
#27306=CARTESIAN_POINT('',(42.196820839876,-72.0466869074717,20.2109458098101));
#27307=CARTESIAN_POINT('Ctrl Pts',(42.196820839876,-72.0466869074717,20.2109458098101));
#27308=CARTESIAN_POINT('Ctrl Pts',(42.1783550388962,-72.3303428376334,20.8234343974591));
#27309=CARTESIAN_POINT('Ctrl Pts',(41.9708816473713,-72.9316905412085,22.1114797855899));
#27310=CARTESIAN_POINT('Ctrl Pts',(41.409110668669,-73.3524778499768,23.2904644816805));
#27311=CARTESIAN_POINT('Ctrl Pts',(41.0736851473658,-73.4473505177094,23.8078632839972));
#27312=CARTESIAN_POINT('Ctrl Pts',(42.2,-71.9490268349807,20.));
#27313=CARTESIAN_POINT('Ctrl Pts',(42.2,-71.9493819426082,20.0007669743775));
#27314=CARTESIAN_POINT('Ctrl Pts',(42.199999888335,-71.9497389941748,20.0015381483622));
#27315=CARTESIAN_POINT('Ctrl Pts',(42.199999576824,-71.9501537653895,20.0024340223005));
#27316=CARTESIAN_POINT('Ctrl Pts',(42.1999992529782,-71.9505849600876,20.0033653697007));
#27317=CARTESIAN_POINT('Ctrl Pts',(42.1999987149955,-71.9510784426047,20.0044312863678));
#27318=CARTESIAN_POINT('Ctrl Pts',(42.1999976675908,-71.9516724317248,20.0057143436616));
#27319=CARTESIAN_POINT('Ctrl Pts',(42.199996568683,-71.9522956285314,20.0070604915641));
#27320=CARTESIAN_POINT('Ctrl Pts',(42.1999949097774,-71.9530293412267,20.0086454048492));
#27321=CARTESIAN_POINT('Ctrl Pts',(42.1999921086958,-71.9538929058103,20.0105108608933));
#27322=CARTESIAN_POINT('Ctrl Pts',(42.1999891261053,-71.954812429029,20.012497197733));
#27323=CARTESIAN_POINT('Ctrl Pts',(42.1999848409495,-71.9558790177824,20.0148012672521));
#27324=CARTESIAN_POINT('Ctrl Pts',(42.1999783277262,-71.9570906515628,20.0174187072715));
#27325=CARTESIAN_POINT('Ctrl Pts',(42.1999711968435,-71.9584171865341,20.0202843633612));
#27326=CARTESIAN_POINT('Ctrl Pts',(42.1999613708697,-71.9599173309903,20.0235251037887));
#27327=CARTESIAN_POINT('Ctrl Pts',(42.1999476265851,-71.9615620166934,20.027078128906));
#27328=CARTESIAN_POINT('Ctrl Pts',(42.1999307119774,-71.9635860735613,20.0314507119941));
#27329=CARTESIAN_POINT('Ctrl Pts',(42.1999077801504,-71.9658285899073,20.0362952820845));
#27330=CARTESIAN_POINT('Ctrl Pts',(42.1998774465528,-71.9682014260206,20.0414214104202));
#27331=CARTESIAN_POINT('Ctrl Pts',(42.1998443239922,-71.9707924278841,20.0470188505451));
#27332=CARTESIAN_POINT('Ctrl Pts',(42.1998023205894,-71.9735361891088,20.0529463298847));
#27333=CARTESIAN_POINT('Ctrl Pts',(42.1997519182532,-71.9763072902013,20.0589328678251));
#27334=CARTESIAN_POINT('Ctrl Pts',(42.1997137069337,-71.9784081338789,20.0634714176514));
#27335=CARTESIAN_POINT('Ctrl Pts',(42.199670746498,-71.9805241019789,20.0680426384819));
#27336=CARTESIAN_POINT('Ctrl Pts',(42.1996239777039,-71.9826126499435,20.0725546053147));
#27337=CARTESIAN_POINT('Ctrl Pts',(42.1995817725225,-71.9844974012468,20.0766263027394));
#27338=CARTESIAN_POINT('Ctrl Pts',(42.1995365022911,-71.9863595591176,20.0806491768695));
#27339=CARTESIAN_POINT('Ctrl Pts',(42.1994888699131,-71.9881839996438,20.0845905429849));
#27340=CARTESIAN_POINT('Ctrl Pts',(42.1994442955512,-71.9898913104193,20.0882788719507));
#27341=CARTESIAN_POINT('Ctrl Pts',(42.1993976796393,-71.9915654195986,20.0918954519325));
#27342=CARTESIAN_POINT('Ctrl Pts',(42.1993491771674,-71.9932117861756,20.0954520617162));
#27343=CARTESIAN_POINT('Ctrl Pts',(42.1993001195776,-71.9948769956621,20.0990493774263));
#27344=CARTESIAN_POINT('Ctrl Pts',(42.1992491686837,-71.9965134300916,20.1025844921456));
#27345=CARTESIAN_POINT('Ctrl Pts',(42.1991955627639,-71.9981501187984,20.106120093224));
#27346=CARTESIAN_POINT('Ctrl Pts',(42.1991432708539,-71.9997466883352,20.1095690282307));
#27347=CARTESIAN_POINT('Ctrl Pts',(42.1990883172282,-72.0013475051531,20.1130270769141));
#27348=CARTESIAN_POINT('Ctrl Pts',(42.1990297058862,-72.0029769497589,20.1165468837949));
#27349=CARTESIAN_POINT('Ctrl Pts',(42.198967654991,-72.0047020168383,20.1202732473384));
#27350=CARTESIAN_POINT('Ctrl Pts',(42.1989014855651,-72.0064590160509,20.1240684967513));
#27351=CARTESIAN_POINT('Ctrl Pts',(42.1988307064682,-72.0082515445906,20.1279403853283));
#27352=CARTESIAN_POINT('Ctrl Pts',(42.1987541012615,-72.0101916233066,20.1321309845027));
#27353=CARTESIAN_POINT('Ctrl Pts',(42.1986720720218,-72.0121730917887,20.136410862965));
#27354=CARTESIAN_POINT('Ctrl Pts',(42.1985851428042,-72.0141745501329,20.1407337874152));
#27355=CARTESIAN_POINT('Ctrl Pts',(42.198483483764,-72.0165151479206,20.1457892148409));
#27356=CARTESIAN_POINT('Ctrl Pts',(42.1983750766135,-72.0188827141844,20.1509027120514));
#27357=CARTESIAN_POINT('Ctrl Pts',(42.198262936023,-72.021212988539,20.1559354939934));
#27358=CARTESIAN_POINT('Ctrl Pts',(42.1980988580267,-72.0246225188898,20.1632991860607));
#27359=CARTESIAN_POINT('Ctrl Pts',(42.1979266789503,-72.0279487284441,20.17048254499));
#27360=CARTESIAN_POINT('Ctrl Pts',(42.1977626383687,-72.0309524054426,20.1769690850139));
#27361=CARTESIAN_POINT('Ctrl Pts',(42.1976578720763,-72.0328707362592,20.1811117839881));
#27362=CARTESIAN_POINT('Ctrl Pts',(42.1975566186956,-72.0346567517583,20.1849686261325));
#27363=CARTESIAN_POINT('Ctrl Pts',(42.1974632723898,-72.0362619872375,20.1884350061837));
#27364=CARTESIAN_POINT('Ctrl Pts',(42.1973769893887,-72.0377457581639,20.1916390930644));
#27365=CARTESIAN_POINT('Ctrl Pts',(42.1972975249792,-72.0390746146824,20.1945085857143));
#27366=CARTESIAN_POINT('Ctrl Pts',(42.1972272050586,-72.040231268269,20.1970061947958));
#27367=CARTESIAN_POINT('Ctrl Pts',(42.1971658233327,-72.0412409024212,20.1991863388396));
#27368=CARTESIAN_POINT('Ctrl Pts',(42.1971114180469,-72.0421193675758,20.2010832152381));
#27369=CARTESIAN_POINT('Ctrl Pts',(42.1970642229353,-72.0428738014203,20.2027122594201));
#27370=CARTESIAN_POINT('Ctrl Pts',(42.197018861125,-72.043598929167,20.2042780231325));
#27371=CARTESIAN_POINT('Ctrl Pts',(42.1969801734843,-72.0442093155135,20.2055960153841));
#27372=CARTESIAN_POINT('Ctrl Pts',(42.1969468971449,-72.0447309293597,20.2067223222945));
#27373=CARTESIAN_POINT('Ctrl Pts',(42.1969151887602,-72.0452279651743,20.2077955585147));
#27374=CARTESIAN_POINT('Ctrl Pts',(42.1968883963498,-72.0456443279215,20.2086945983907));
#27375=CARTESIAN_POINT('Ctrl Pts',(42.1968639639419,-72.0460222101615,20.2095105488797));
#27376=CARTESIAN_POINT('Ctrl Pts',(42.1968490294804,-72.0462531930326,20.2100093036948));
#27377=CARTESIAN_POINT('Ctrl Pts',(42.1968349481487,-72.0464701881852,20.2104778552371));
#27378=CARTESIAN_POINT('Ctrl Pts',(42.196820839876,-72.0466869074717,20.2109458098101));
#27379=CARTESIAN_POINT('Ctrl Pts',(-4.59286786251854,-72.9498130615488,
-26.9309675781303));
#27380=CARTESIAN_POINT('Ctrl Pts',(-4.58597883112302,-72.9467708226897,
-26.9319238812612));
#27381=CARTESIAN_POINT('Ctrl Pts',(-4.57152330186566,-72.9403541543873,
-26.9337973859128));
#27382=CARTESIAN_POINT('Ctrl Pts',(-4.48780388137234,-72.9035146304749,
-26.9456499185224));
#27383=CARTESIAN_POINT('Ctrl Pts',(-4.23649589071421,-72.7907458248883,
-26.9734457827405));
#27384=CARTESIAN_POINT('Ctrl Pts',(-3.96644514618002,-72.665579126758,-26.9924939495254));
#27385=CARTESIAN_POINT('Ctrl Pts',(-3.71514557682102,-72.548594622924,-27.0001369004246));
#27386=CARTESIAN_POINT('Ctrl Pts',(-3.63119107772806,-72.5097909109609,
-26.9998430869986));
#27387=CARTESIAN_POINT('Ctrl Pts',(-3.61668235972474,-72.5031611812015,
-27.));
#27388=CARTESIAN_POINT('Ctrl Pts',(-3.60976192857618,-72.5,-27.));
#27389=CARTESIAN_POINT('Ctrl Pts',(-4.73222628093364,-72.6487705946061,
-26.9529186924327));
#27390=CARTESIAN_POINT('Ctrl Pts',(-4.72712574225606,-72.6464928862309,
-26.9533741257428));
#27391=CARTESIAN_POINT('Ctrl Pts',(-4.71810316556283,-72.6424665759273,
-26.9541650696995));
#27392=CARTESIAN_POINT('Ctrl Pts',(-4.66022923522091,-72.6172314047933,
-26.9623845226138));
#27393=CARTESIAN_POINT('Ctrl Pts',(-4.46228371256307,-72.5287892895904,
-26.9851096971082));
#27394=CARTESIAN_POINT('Ctrl Pts',(-4.27646988143267,-72.442180089981,-26.9974869463342));
#27395=CARTESIAN_POINT('Ctrl Pts',(-4.07861559516288,-72.3497082397124,
-27.0015613961821));
#27396=CARTESIAN_POINT('Ctrl Pts',(-4.02063676120937,-72.3228011601093,
-26.9999955597789));
#27397=CARTESIAN_POINT('Ctrl Pts',(-4.01161227485084,-72.3186769260278,
-27.));
#27398=CARTESIAN_POINT('Ctrl Pts',(-4.00650795238412,-72.3163422783269,
-27.));
#27399=CARTESIAN_POINT('Ctrl Pts',(-4.87158469934875,-72.3477281276634,
-26.9748698067351));
#27400=CARTESIAN_POINT('Ctrl Pts',(-4.86830808893293,-72.346245599186,-26.9750197376998));
#27401=CARTESIAN_POINT('Ctrl Pts',(-4.85975975168661,-72.3423622412983,
-26.9755924149209));
#27402=CARTESIAN_POINT('Ctrl Pts',(-4.81588843551312,-72.3223172404505,
-26.9789296879549));
#27403=CARTESIAN_POINT('Ctrl Pts',(-4.70844366796589,-72.2729883046416,
-26.9857195731902));
#27404=CARTESIAN_POINT('Ctrl Pts',(-4.56627474372858,-72.2076842290428,
-26.9947091274986));
#27405=CARTESIAN_POINT('Ctrl Pts',(-4.45897436459025,-72.1582939535662,
-26.9983929926645));
#27406=CARTESIAN_POINT('Ctrl Pts',(-4.41510722369007,-72.138122645422,-26.999758423857));
#27407=CARTESIAN_POINT('Ctrl Pts',(-4.40654218997694,-72.1341926708542,
-27.));
#27408=CARTESIAN_POINT('Ctrl Pts',(-4.40325397619206,-72.1326845566538,
-27.));
#27409=CARTESIAN_POINT('Ctrl Pts',(-5.01094311776385,-72.0466856607207,
-26.9968209210375));
#27410=CARTESIAN_POINT('Ctrl Pts',(-5.00947183604093,-72.0460042802039,
-26.9968652778614));
#27411=CARTESIAN_POINT('Ctrl Pts',(-5.00638341486692,-72.0445740412427,
-26.9969519897208));
#27412=CARTESIAN_POINT('Ctrl Pts',(-4.98844404444095,-72.0362656438942,
-26.9975053631966));
#27413=CARTESIAN_POINT('Ctrl Pts',(-4.93447171373018,-72.0112738204271,
-26.9987930811475));
#27414=CARTESIAN_POINT('Ctrl Pts',(-4.87648104575523,-71.9844301094941,
-26.9996559735758));
#27415=CARTESIAN_POINT('Ctrl Pts',(-4.8225217894526,-71.959453134982,-27.0000061189091));
#27416=CARTESIAN_POINT('Ctrl Pts',(-4.80456005745059,-71.9511381192262,
-26.9999927847699));
#27417=CARTESIAN_POINT('Ctrl Pts',(-4.80147210510304,-71.9497084156806,
-27.));
#27418=CARTESIAN_POINT('Ctrl Pts',(-4.8,-71.9490268349807,-27.));
#27419=CARTESIAN_POINT('',(-4.59286786251854,-72.9498130615488,-26.9309675781303));
#27420=CARTESIAN_POINT('Ctrl Pts',(-3.60976192857618,-72.5,-27.));
#27421=CARTESIAN_POINT('Ctrl Pts',(-3.6121798317656,-72.5011044731095,-27.));
#27422=CARTESIAN_POINT('Ctrl Pts',(-3.61460175619875,-72.5022108180881,
-26.9999988447398));
#27423=CARTESIAN_POINT('Ctrl Pts',(-3.61720808063408,-72.5034032651581,
-26.9999961392571));
#27424=CARTESIAN_POINT('Ctrl Pts',(-3.61987818981872,-72.5046248950636,
-26.999993367563));
#27425=CARTESIAN_POINT('Ctrl Pts',(-3.62274171103015,-72.5059368360811,
-26.9999889713356));
#27426=CARTESIAN_POINT('Ctrl Pts',(-3.62594300170539,-72.5074065633977,
-26.9999817141614));
#27427=CARTESIAN_POINT('Ctrl Pts',(-3.6292333827049,-72.5089171924931,-26.9999742550237));
#27428=CARTESIAN_POINT('Ctrl Pts',(-3.63288045211659,-72.5105944472574,
-26.9999637812448));
#27429=CARTESIAN_POINT('Ctrl Pts',(-3.63699121203846,-72.5124884140809,
-26.9999480122703));
#27430=CARTESIAN_POINT('Ctrl Pts',(-3.64123459139212,-72.5144434831845,
-26.9999317345645));
#27431=CARTESIAN_POINT('Ctrl Pts',(-3.64597189527866,-72.5166293969509,
-26.9999098171331));
#27432=CARTESIAN_POINT('Ctrl Pts',(-3.65127087672114,-72.5190779485736,
-26.9998786723859));
#27433=CARTESIAN_POINT('Ctrl Pts',(-3.65689722795564,-72.5216777711234,
-26.9998456035239));
#27434=CARTESIAN_POINT('Ctrl Pts',(-3.66315677356868,-72.5245736760054,
-26.9998021229674));
#27435=CARTESIAN_POINT('Ctrl Pts',(-3.67007637899193,-72.5277783735898,
-26.9997427652637));
#27436=CARTESIAN_POINT('Ctrl Pts',(-3.67736092134016,-72.5311520855053,
-26.9996802770609));
#27437=CARTESIAN_POINT('Ctrl Pts',(-3.68537672523341,-72.5348679050117,
-26.9996001514933));
#27438=CARTESIAN_POINT('Ctrl Pts',(-3.69409908715974,-72.538914401124,-26.9994951381666));
#27439=CARTESIAN_POINT('Ctrl Pts',(-3.70344137655423,-72.5432484952644,
-26.9993826611911));
#27440=CARTESIAN_POINT('Ctrl Pts',(-3.71359387467642,-72.5479617814959,
-26.9992415459466));
#27441=CARTESIAN_POINT('Ctrl Pts',(-3.7244680994068,-72.5530128872099,-26.999062918556));
#27442=CARTESIAN_POINT('Ctrl Pts',(-3.7365221810632,-72.5586120395395,-26.9988649100353));
#27443=CARTESIAN_POINT('Ctrl Pts',(-3.74946252996333,-72.5646260341567,
-26.9986206326566));
#27444=CARTESIAN_POINT('Ctrl Pts',(-3.76310633289472,-72.5709691128928,
-26.9983201877487));
#27445=CARTESIAN_POINT('Ctrl Pts',(-3.77980856865807,-72.5787340738093,
-26.9979523942741));
#27446=CARTESIAN_POINT('Ctrl Pts',(-3.79756346992481,-72.5869914895461,
-26.9974999166189));
#27447=CARTESIAN_POINT('Ctrl Pts',(-3.815960640567,-72.5955484292695,-26.99695373932));
#27448=CARTESIAN_POINT('Ctrl Pts',(-3.83486113114969,-72.604339474469,-26.9963926194013));
#27449=CARTESIAN_POINT('Ctrl Pts',(-3.85443398804955,-72.6134440505967,
-26.9957325028426));
#27450=CARTESIAN_POINT('Ctrl Pts',(-3.87422314146776,-72.6226474512837,
-26.9949774589249));
#27451=CARTESIAN_POINT('Ctrl Pts',(-3.89002366524084,-72.6299958480683,
-26.9943745989077));
#27452=CARTESIAN_POINT('Ctrl Pts',(-3.90596073606572,-72.6374066137615,
-26.9937116122647));
#27453=CARTESIAN_POINT('Ctrl Pts',(-3.92183420187478,-72.644785372869,-26.9929960468143));
#27454=CARTESIAN_POINT('Ctrl Pts',(-3.93600161067149,-72.6513710736823,
-26.9923573892975));
#27455=CARTESIAN_POINT('Ctrl Pts',(-3.95011786238888,-72.6579310555987,
-26.9916770268006));
#27456=CARTESIAN_POINT('Ctrl Pts',(-3.96407960253109,-72.6644163574739,
-26.9909618577935));
#27457=CARTESIAN_POINT('Ctrl Pts',(-3.97708743249592,-72.6704585630446,
-26.9902955513915));
#27458=CARTESIAN_POINT('Ctrl Pts',(-3.98996081458732,-72.676435800597,-26.9895991550418));
#27459=CARTESIAN_POINT('Ctrl Pts',(-4.00265755428967,-72.6823276467238,
-26.9888776407886));
#27460=CARTESIAN_POINT('Ctrl Pts',(-4.01471371198153,-72.6879222345996,
-26.988192528719));
#27461=CARTESIAN_POINT('Ctrl Pts',(-4.02661035498069,-72.6934397254355,
-26.9874848652863));
#27462=CARTESIAN_POINT('Ctrl Pts',(-4.03835411814552,-72.6988823143548,
-26.986756814357));
#27463=CARTESIAN_POINT('Ctrl Pts',(-4.0496271379236,-72.7041067395813,-26.9860579470169));
#27464=CARTESIAN_POINT('Ctrl Pts',(-4.06075909094922,-72.7092620662293,
-26.9853403733249));
#27465=CARTESIAN_POINT('Ctrl Pts',(-4.07179949547093,-72.7143701921724,
-26.9846027821299));
#27466=CARTESIAN_POINT('Ctrl Pts',(-4.08305161322444,-72.7195762726651,
-26.9838510467236));
#27467=CARTESIAN_POINT('Ctrl Pts',(-4.09420802299186,-72.7247330573131,
-26.9830786440317));
#27468=CARTESIAN_POINT('Ctrl Pts',(-4.10537436234696,-72.729887888526,-26.9822791770477));
#27469=CARTESIAN_POINT('Ctrl Pts',(-4.11610685214918,-72.7348424373415,
-26.9815107720242));
#27470=CARTESIAN_POINT('Ctrl Pts',(-4.12685642878814,-72.7397987793188,
-26.9807167793448));
#27471=CARTESIAN_POINT('Ctrl Pts',(-4.13770638415419,-72.7447940225878,
-26.9798904981468));
#27472=CARTESIAN_POINT('Ctrl Pts',(-4.14894230031643,-72.7499669594974,
-26.9790348240032));
#27473=CARTESIAN_POINT('Ctrl Pts',(-4.16028567191421,-72.755181518857,-26.9781444707583));
#27474=CARTESIAN_POINT('Ctrl Pts',(-4.17177856524463,-72.7604559078795,
-26.9772145138912));
#27475=CARTESIAN_POINT('Ctrl Pts',(-4.1840671780142,-72.7660954733422,-26.9762201707346));
#27476=CARTESIAN_POINT('Ctrl Pts',(-4.19652668861544,-72.771803406091,-26.9751804717657));
#27477=CARTESIAN_POINT('Ctrl Pts',(-4.20915332155542,-72.7775769562583,
-26.974093291944));
#27478=CARTESIAN_POINT('Ctrl Pts',(-4.2225448421669,-72.7837002526615,-26.9729402536749));
#27479=CARTESIAN_POINT('Ctrl Pts',(-4.23612401933091,-72.7898971879111,
-26.9717337257237));
#27480=CARTESIAN_POINT('Ctrl Pts',(-4.24982926006434,-72.7961388946508,
-26.9704767101437));
#27481=CARTESIAN_POINT('Ctrl Pts',(-4.26471116374373,-72.8029164828962,
-26.9691117735367));
#27482=CARTESIAN_POINT('Ctrl Pts',(-4.27974121837608,-72.809746603987,-26.967687199763));
#27483=CARTESIAN_POINT('Ctrl Pts',(-4.2947812708956,-72.8165662126102,-26.9662147977134));
#27484=CARTESIAN_POINT('Ctrl Pts',(-4.31217847082007,-72.8244546222066,
-26.964511633925));
#27485=CARTESIAN_POINT('Ctrl Pts',(-4.32958814165081,-72.8323284779439,
-26.9627442813405));
#27486=CARTESIAN_POINT('Ctrl Pts',(-4.34673013421309,-72.8400621253335,
-26.9609441299768));
#27487=CARTESIAN_POINT('Ctrl Pts',(-4.36908646666351,-72.8501482335539,
-26.958596399268));
#27488=CARTESIAN_POINT('Ctrl Pts',(-4.3909822100646,-72.8599932152661,-26.9561926445271));
#27489=CARTESIAN_POINT('Ctrl Pts',(-4.41173359126681,-72.8692963615835,
-26.9538294938958));
#27490=CARTESIAN_POINT('Ctrl Pts',(-4.42638773343343,-72.87586602687,-26.9521606919508));
#27491=CARTESIAN_POINT('Ctrl Pts',(-4.44046920811496,-72.882164767821,-26.9505129508519));
#27492=CARTESIAN_POINT('Ctrl Pts',(-4.45375849835115,-72.8880981139709,
-26.9489236880982));
#27493=CARTESIAN_POINT('Ctrl Pts',(-4.46568249135964,-72.8934218879838,
-26.947497700884));
#27494=CARTESIAN_POINT('Ctrl Pts',(-4.47696801229591,-72.8984512256794,
-26.9461190319865));
#27495=CARTESIAN_POINT('Ctrl Pts',(-4.4874906704524,-72.9031338368651,-26.9448124824954));
#27496=CARTESIAN_POINT('Ctrl Pts',(-4.49731427885776,-72.9075053690311,
-26.9435927307584));
#27497=CARTESIAN_POINT('Ctrl Pts',(-4.50647257936972,-72.9115745492459,
-26.9424359792803));
#27498=CARTESIAN_POINT('Ctrl Pts',(-4.51490348064674,-72.9153163971461,
-26.9413577939781));
#27499=CARTESIAN_POINT('Ctrl Pts',(-4.52291802255619,-72.918873454195,-26.9403328547686));
#27500=CARTESIAN_POINT('Ctrl Pts',(-4.53027491933034,-72.9221345908914,
-26.939379007774));
#27501=CARTESIAN_POINT('Ctrl Pts',(-4.53696273809178,-72.9250967827365,
-26.9385036410476));
#27502=CARTESIAN_POINT('Ctrl Pts',(-4.54338726026832,-72.9279423543464,
-26.9376627371375));
#27503=CARTESIAN_POINT('Ctrl Pts',(-4.54919410148017,-72.9305119583038,
-26.9368943156625));
#27504=CARTESIAN_POINT('Ctrl Pts',(-4.55441685885851,-72.932821936876,-26.93619816563));
#27505=CARTESIAN_POINT('Ctrl Pts',(-4.55939180148987,-72.9350223092165,
-26.9355350472379));
#27506=CARTESIAN_POINT('Ctrl Pts',(-4.56383669313756,-72.9369870780139,
-26.9349375205309));
#27507=CARTESIAN_POINT('Ctrl Pts',(-4.56782323678299,-72.9387488347678,
-26.9343986405424));
#27508=CARTESIAN_POINT('Ctrl Pts',(-4.5717196612956,-72.9404707655458,-26.933871942384));
#27509=CARTESIAN_POINT('Ctrl Pts',(-4.57517802327509,-72.9419986707184,
-26.9334012948219));
#27510=CARTESIAN_POINT('Ctrl Pts',(-4.57830933875514,-72.9433820368179,
-26.9329732619373));
#27511=CARTESIAN_POINT('Ctrl Pts',(-4.58134224987413,-72.9447219294131,
-26.932558680365));
#27512=CARTESIAN_POINT('Ctrl Pts',(-4.58406826147243,-72.9459261859508,
-26.9321840818725));
#27513=CARTESIAN_POINT('Ctrl Pts',(-4.58663203070186,-72.9470587250243,
-26.9318304705445));
#27514=CARTESIAN_POINT('Ctrl Pts',(-4.58878734423874,-72.9480108297488,
-26.9315331960186));
#27515=CARTESIAN_POINT('Ctrl Pts',(-4.59082864516527,-72.9489125305571,
-26.9312506527496));
#27516=CARTESIAN_POINT('Ctrl Pts',(-4.59286786251854,-72.9498130615488,
-26.9309675781303));
#27517=CARTESIAN_POINT('',(-5.01094311776385,-72.0466856607207,-26.9968209210375));
#27518=CARTESIAN_POINT('Ctrl Pts',(-5.01094311776385,-72.0466856607207,
-26.9968209210375));
#27519=CARTESIAN_POINT('Ctrl Pts',(-4.87158469934875,-72.3477281276634,
-26.9748698067351));
#27520=CARTESIAN_POINT('Ctrl Pts',(-4.73222628093364,-72.6487705946061,
-26.9529186924327));
#27521=CARTESIAN_POINT('Ctrl Pts',(-4.59286786251854,-72.9498130615488,
-26.9309675781303));
#27522=CARTESIAN_POINT('Ctrl Pts',(-5.01094311776385,-72.0466856607207,
-26.9968209210375));
#27523=CARTESIAN_POINT('Ctrl Pts',(-5.01017656486953,-72.0463306544706,
-26.9968440313985));
#27524=CARTESIAN_POINT('Ctrl Pts',(-5.00940581101761,-72.0459737040594,
-26.9968671567182));
#27525=CARTESIAN_POINT('Ctrl Pts',(-5.00851041310935,-72.0455590281858,
-26.9968938399568));
#27526=CARTESIAN_POINT('Ctrl Pts',(-5.00757955946722,-72.0451279320846,
-26.9969215797913));
#27527=CARTESIAN_POINT('Ctrl Pts',(-5.00651419661325,-72.0446345417407,
-26.9969531606685));
#27528=CARTESIAN_POINT('Ctrl Pts',(-5.00523178583954,-72.0440406347171,
-26.9969907756178));
#27529=CARTESIAN_POINT('Ctrl Pts',(-5.00388631377784,-72.0434175229001,
-26.9970302402453));
#27530=CARTESIAN_POINT('Ctrl Pts',(-5.00230217741908,-72.0426838837101,
-26.9970763400509));
#27531=CARTESIAN_POINT('Ctrl Pts',(-5.00043760367473,-72.041820379669,-26.9971297520507));
#27532=CARTESIAN_POINT('Ctrl Pts',(-4.99845220009132,-72.0409009180372,
-26.9971866253046));
#27533=CARTESIAN_POINT('Ctrl Pts',(-4.9961491809407,-72.0398343752721,-26.9972517711657));
#27534=CARTESIAN_POINT('Ctrl Pts',(-4.99353288021377,-72.0386227730732,
-26.9973241331438));
#27535=CARTESIAN_POINT('Ctrl Pts',(-4.99066845283999,-72.0372962640566,
-26.9974033578401));
#27536=CARTESIAN_POINT('Ctrl Pts',(-4.98742904190035,-72.0357961260636,
-26.9974911916518));
#27537=CARTESIAN_POINT('Ctrl Pts',(-4.98387738276555,-72.0341514325883,
-26.9975845195401));
#27538=CARTESIAN_POINT('Ctrl Pts',(-4.97950627706432,-72.0321272718358,
-26.9976993802429));
#27539=CARTESIAN_POINT('Ctrl Pts',(-4.97466319276724,-72.0298846097017,
-26.9978224504092));
#27540=CARTESIAN_POINT('Ctrl Pts',(-4.96953845441555,-72.02751161209,-26.9979466068608));
#27541=CARTESIAN_POINT('Ctrl Pts',(-4.96394341208111,-72.0249208413646,
-26.9980821573134));
#27542=CARTESIAN_POINT('Ctrl Pts',(-4.95801831699475,-72.0221773413901,
-26.998218776321));
#27543=CARTESIAN_POINT('Ctrl Pts',(-4.952033932691,-72.0194065054176,-26.998348782628));
#27544=CARTESIAN_POINT('Ctrl Pts',(-4.94749666544916,-72.0173057006142,
-26.998447351391));
#27545=CARTESIAN_POINT('Ctrl Pts',(-4.94292659089731,-72.0151897711979,
-26.998542158666));
#27546=CARTESIAN_POINT('Ctrl Pts',(-4.93841559860224,-72.0131012617228,
-26.9986313749235));
#27547=CARTESIAN_POINT('Ctrl Pts',(-4.93434475476635,-72.0112165331827,
-26.9987118861344));
#27548=CARTESIAN_POINT('Ctrl Pts',(-4.93032259575766,-72.0093543982208,
-26.9987878633368));
#27549=CARTESIAN_POINT('Ctrl Pts',(-4.92638179739851,-72.0075299799368,
-26.9988590242472));
#27550=CARTESIAN_POINT('Ctrl Pts',(-4.92269399034503,-72.0058226856267,
-26.9989256167707));
#27551=CARTESIAN_POINT('Ctrl Pts',(-4.91907780420724,-72.0041485925123,
-26.99898800739));
#27552=CARTESIAN_POINT('Ctrl Pts',(-4.91552145808714,-72.0025022394493,
-26.9990467059966));
#27553=CARTESIAN_POINT('Ctrl Pts',(-4.91192336677503,-72.0008365611231,
-26.9991060936207));
#27554=CARTESIAN_POINT('Ctrl Pts',(-4.90838738253759,-71.9991996731572,
-26.9991617130831));
#27555=CARTESIAN_POINT('Ctrl Pts',(-4.90485074937926,-71.9975625131326,
-26.9992146931177));
#27556=CARTESIAN_POINT('Ctrl Pts',(-4.90140179900313,-71.9959659427703,
-26.9992663596328));
#27557=CARTESIAN_POINT('Ctrl Pts',(-4.89794358042941,-71.994365108323,-26.9993156414398));
#27558=CARTESIAN_POINT('Ctrl Pts',(-4.89442346735378,-71.9927356391644,
-26.9993631288006));
#27559=CARTESIAN_POINT('Ctrl Pts',(-4.89069675220022,-71.9910105333865,
-26.9994134032841));
#27560=CARTESIAN_POINT('Ctrl Pts',(-4.88690099672145,-71.9892534872454,
-26.9994616375389));
#27561=CARTESIAN_POINT('Ctrl Pts',(-4.88302846534461,-71.9874609128104,
-26.9995075736756));
#27562=CARTESIAN_POINT('Ctrl Pts',(-4.87883711126807,-71.9855207570222,
-26.9995572917012));
#27563=CARTESIAN_POINT('Ctrl Pts',(-4.87455631436082,-71.983539211521,-26.9996042784301));
#27564=CARTESIAN_POINT('Ctrl Pts',(-4.87023234098015,-71.9815376862609,
-26.9996476638671));
#27565=CARTESIAN_POINT('Ctrl Pts',(-4.86517549990667,-71.9791969236675,
-26.9996984026762));
#27566=CARTESIAN_POINT('Ctrl Pts',(-4.86006040492235,-71.9768292045297,
-26.9997441449775));
#27567=CARTESIAN_POINT('Ctrl Pts',(-4.85502594174055,-71.9744988084778,
-26.9997837213542));
#27568=CARTESIAN_POINT('Ctrl Pts',(-4.84766089691437,-71.9710896125487,
-26.999841618647));
#27569=CARTESIAN_POINT('Ctrl Pts',(-4.84047595262308,-71.9677637815372,
-26.9998859843948));
#27570=CARTESIAN_POINT('Ctrl Pts',(-4.83398778844191,-71.9647604551997,
-26.9999174873878));
#27571=CARTESIAN_POINT('Ctrl Pts',(-4.82984402883823,-71.9628423375308,
-26.9999376072285));
#27572=CARTESIAN_POINT('Ctrl Pts',(-4.82598611616407,-71.9610565242511,
-26.9999526244651));
#27573=CARTESIAN_POINT('Ctrl Pts',(-4.82251871585362,-71.9594514605147,
-26.9999637790089));
#27574=CARTESIAN_POINT('Ctrl Pts',(-4.81931370885316,-71.9579678589542,
-26.9999740894397));
#27575=CARTESIAN_POINT('Ctrl Pts',(-4.81644333517054,-71.9566391432613,
-26.9999811327487));
#27576=CARTESIAN_POINT('Ctrl Pts',(-4.8139449187002,-71.9554825904982,-26.9999861099321));
#27577=CARTESIAN_POINT('Ctrl Pts',(-4.81176395371457,-71.9544729905736,
-26.9999904547092));
#27578=CARTESIAN_POINT('Ctrl Pts',(-4.80986634322754,-71.9535945432726,
-26.9999932365079));
#27579=CARTESIAN_POINT('Ctrl Pts',(-4.80823665587008,-71.9528401072577,
-26.9999951541055));
#27580=CARTESIAN_POINT('Ctrl Pts',(-4.80667026905868,-71.9521149751527,
-26.9999969972195));
#27581=CARTESIAN_POINT('Ctrl Pts',(-4.80535173946758,-71.95150456664,-26.9999980448942));
#27582=CARTESIAN_POINT('Ctrl Pts',(-4.80422495748871,-71.9509829115286,
-26.9999987249809));
#27583=CARTESIAN_POINT('Ctrl Pts',(-4.80315126323157,-71.9504858339149,
-26.9999993730257));
#27584=CARTESIAN_POINT('Ctrl Pts',(-4.80225182361175,-71.9500694128276,
-26.9999996854072));
#27585=CARTESIAN_POINT('Ctrl Pts',(-4.80143548384865,-71.9496914561439,
-26.9999998528133));
#27586=CARTESIAN_POINT('Ctrl Pts',(-4.80093666763287,-71.9494605095072,
-26.9999999551051));
#27587=CARTESIAN_POINT('Ctrl Pts',(-4.80046803628928,-71.9492435345227,
-27.));
#27588=CARTESIAN_POINT('Ctrl Pts',(-4.8,-71.9490268349807,-27.));
#27589=CARTESIAN_POINT('Ctrl Pts',(-11.7968208397773,-72.0466869089798,
-20.2109458130836));
#27590=CARTESIAN_POINT('Ctrl Pts',(-11.7968651976611,-72.0460055208926,
-20.2094745150254));
#27591=CARTESIAN_POINT('Ctrl Pts',(-11.7969519115959,-72.0445752658204,
-20.2063860590447));
#27592=CARTESIAN_POINT('Ctrl Pts',(-11.7975052989931,-72.0362667659614,
-20.188446468735));
#27593=CARTESIAN_POINT('Ctrl Pts',(-11.7987930505529,-72.011274612559,-20.1344734253031));
#27594=CARTESIAN_POINT('Ctrl Pts',(-11.7996559651957,-71.9844305551918,
-20.0764819862767));
#27595=CARTESIAN_POINT('Ctrl Pts',(-11.8000061190643,-71.9594532702652,
-20.0225220618368));
#27596=CARTESIAN_POINT('Ctrl Pts',(-11.7999927845943,-71.9511381475697,
-20.0045601118682));
#27597=CARTESIAN_POINT('Ctrl Pts',(-11.8,-71.9497084248729,-20.0014721226545));
#27598=CARTESIAN_POINT('Ctrl Pts',(-11.8,-71.9490268349807,-20.));
#27599=CARTESIAN_POINT('Ctrl Pts',(-11.7748696277249,-72.3477293569724,
-20.0715873955272));
#27600=CARTESIAN_POINT('Ctrl Pts',(-11.775019560245,-72.3462468306403,-20.0683107896909));
#27601=CARTESIAN_POINT('Ctrl Pts',(-11.7755113158618,-72.3423634681059,
-20.059760561131));
#27602=CARTESIAN_POINT('Ctrl Pts',(-11.7782701110629,-72.3223183598903,
-20.0159147531201));
#27603=CARTESIAN_POINT('Ctrl Pts',(-11.7845160683301,-72.272988998898,-19.9085744635702));
#27604=CARTESIAN_POINT('Ctrl Pts',(-11.793098520739,-72.2076844580308,-19.7663907236395));
#27605=CARTESIAN_POINT('Ctrl Pts',(-11.7980897330917,-72.1582938607934,
-19.6590311388775));
#27606=CARTESIAN_POINT('Ctrl Pts',(-11.7997839095829,-72.1381225726863,
-19.6151120373436));
#27607=CARTESIAN_POINT('Ctrl Pts',(-11.8,-72.1341926423671,-19.6065422105488));
#27608=CARTESIAN_POINT('Ctrl Pts',(-11.8,-72.1326845566538,-19.6032539761921));
#27609=CARTESIAN_POINT('Ctrl Pts',(-11.7529184156725,-72.6487718049651,
-19.9322289779709));
#27610=CARTESIAN_POINT('Ctrl Pts',(-11.7533738483013,-72.6464941083948,
-19.9271284649557));
#27611=CARTESIAN_POINT('Ctrl Pts',(-11.7544900684487,-72.6425809301834,
-19.9181059391757));
#27612=CARTESIAN_POINT('Ctrl Pts',(-11.7622980156172,-72.615950659827,-19.860231931054));
#27613=CARTESIAN_POINT('Ctrl Pts',(-11.7782324373171,-72.5231684604105,
-19.6622853069392));
#27614=CARTESIAN_POINT('Ctrl Pts',(-11.7937561910005,-72.4384015726793,
-19.4764707261542));
#27615=CARTESIAN_POINT('Ctrl Pts',(-11.7979643479897,-72.3480969257325,
-19.2786158960547));
#27616=CARTESIAN_POINT('Ctrl Pts',(-11.7994070877583,-72.3226741083817,
-19.2206368296666));
#27617=CARTESIAN_POINT('Ctrl Pts',(-11.8,-72.3186768598613,-19.2116122984431));
#27618=CARTESIAN_POINT('Ctrl Pts',(-11.8,-72.3163422783269,-19.2065079523841));
#27619=CARTESIAN_POINT('Ctrl Pts',(-11.73096720362,-72.9498142529578,-19.7928705604145));
#27620=CARTESIAN_POINT('Ctrl Pts',(-11.7319235028288,-72.94677203543,-19.7859815754942));
#27621=CARTESIAN_POINT('Ctrl Pts',(-11.7337970013036,-72.9403554050036,
-19.7715261332556));
#27622=CARTESIAN_POINT('Ctrl Pts',(-11.7456495505882,-72.9035159512033,
-19.687806713427));
#27623=CARTESIAN_POINT('Ctrl Pts',(-11.7734456662866,-72.7907466259382,
-19.4364976352758));
#27624=CARTESIAN_POINT('Ctrl Pts',(-11.7924940627946,-72.6655783935656,
-19.1664460935647));
#27625=CARTESIAN_POINT('Ctrl Pts',(-11.8001369169024,-72.5485937708681,
-18.9151459228174));
#27626=CARTESIAN_POINT('Ctrl Pts',(-11.7998430886325,-72.5097906048016,
-18.8311911573673));
#27627=CARTESIAN_POINT('Ctrl Pts',(-11.8,-72.5031610773555,-18.8166823863373));
#27628=CARTESIAN_POINT('Ctrl Pts',(-11.8,-72.5,-18.8097619285762));
#27629=CARTESIAN_POINT('',(-11.8,-71.9490268349807,-20.));
#27630=CARTESIAN_POINT('',(-11.7968208397773,-72.0466869089798,-20.2109458130836));
#27631=CARTESIAN_POINT('Ctrl Pts',(-11.8,-71.9490268349807,-20.));
#27632=CARTESIAN_POINT('Ctrl Pts',(-11.8,-71.9493819426124,-20.0007669743864));
#27633=CARTESIAN_POINT('Ctrl Pts',(-11.799999888335,-71.9497389941831,-20.0015381483801));
#27634=CARTESIAN_POINT('Ctrl Pts',(-11.7999995768239,-71.9501537654007,
-20.0024340223285));
#27635=CARTESIAN_POINT('Ctrl Pts',(-11.7999992529781,-71.950584960102,-20.003365369739));
#27636=CARTESIAN_POINT('Ctrl Pts',(-11.7999987149954,-71.9510784426209,
-20.0044312864177));
#27637=CARTESIAN_POINT('Ctrl Pts',(-11.7999976675907,-71.9516724317409,
-20.0057143437254));
#27638=CARTESIAN_POINT('Ctrl Pts',(-11.799996568683,-71.9522956285472,-20.0070604916421));
#27639=CARTESIAN_POINT('Ctrl Pts',(-11.7999949097773,-71.9530293412399,
-20.008645404944));
#27640=CARTESIAN_POINT('Ctrl Pts',(-11.7999921086956,-71.9538929058181,
-20.0105108610082));
#27641=CARTESIAN_POINT('Ctrl Pts',(-11.799989126105,-71.9548124290305,-20.0124971978685));
#27642=CARTESIAN_POINT('Ctrl Pts',(-11.7999848409491,-71.9558790177743,
-20.0148012674117));
#27643=CARTESIAN_POINT('Ctrl Pts',(-11.7999783277258,-71.9570906515413,
-20.0174187074598));
#27644=CARTESIAN_POINT('Ctrl Pts',(-11.7999711968429,-71.958417186497,-20.0202843635784));
#27645=CARTESIAN_POINT('Ctrl Pts',(-11.7999613708689,-71.9599173309328,
-20.0235251040395));
#27646=CARTESIAN_POINT('Ctrl Pts',(-11.799947626584,-71.9615620166113,-20.0270781291961));
#27647=CARTESIAN_POINT('Ctrl Pts',(-11.799930711976,-71.963586073436,-20.0314507123044));
#27648=CARTESIAN_POINT('Ctrl Pts',(-11.7999077801487,-71.9658285897296,
-20.0362952824175));
#27649=CARTESIAN_POINT('Ctrl Pts',(-11.7998774465507,-71.9682014257852,
-20.0414214107826));
#27650=CARTESIAN_POINT('Ctrl Pts',(-11.7998443239889,-71.9707924276407,
-20.0470188510583));
#27651=CARTESIAN_POINT('Ctrl Pts',(-11.7998023205844,-71.9735361888576,
-20.052946330571));
#27652=CARTESIAN_POINT('Ctrl Pts',(-11.7997519182459,-71.9763072899415,
-20.0589328686926));
#27653=CARTESIAN_POINT('Ctrl Pts',(-11.7997137069251,-71.9784081335907,
-20.0634714186095));
#27654=CARTESIAN_POINT('Ctrl Pts',(-11.7996707464879,-71.9805241016616,
-20.0680426395345));
#27655=CARTESIAN_POINT('Ctrl Pts',(-11.799623977692,-71.9826126495981,-20.0725546064623));
#27656=CARTESIAN_POINT('Ctrl Pts',(-11.7995817725091,-71.9844974008745,
-20.0766263039694));
#27657=CARTESIAN_POINT('Ctrl Pts',(-11.799536502276,-71.9863595587191,-20.0806491781825));
#27658=CARTESIAN_POINT('Ctrl Pts',(-11.7994888698963,-71.9881839992219,
-20.0845905443789));
#27659=CARTESIAN_POINT('Ctrl Pts',(-11.7994442955327,-71.989891309975,-20.0882788734193));
#27660=CARTESIAN_POINT('Ctrl Pts',(-11.7993976796191,-71.9915654191343,
-20.0918954534738));
#27661=CARTESIAN_POINT('Ctrl Pts',(-11.7993491771455,-71.9932117856955,
-20.0954520633262));
#27662=CARTESIAN_POINT('Ctrl Pts',(-11.7993001195565,-71.9948769950761,
-20.0990493789115));
#27663=CARTESIAN_POINT('Ctrl Pts',(-11.7992491686637,-71.9965134294075,
-20.102584493509));
#27664=CARTESIAN_POINT('Ctrl Pts',(-11.7991955627453,-71.9981501180208,
-20.1061200944543));
#27665=CARTESIAN_POINT('Ctrl Pts',(-11.7991432708341,-71.9997466875428,
-20.1095690294963));
#27666=CARTESIAN_POINT('Ctrl Pts',(-11.7990883172074,-72.0013475043506,
-20.1130270782043));
#27667=CARTESIAN_POINT('Ctrl Pts',(-11.7990297058644,-72.0029769489546,
-20.1165468851023));
#27668=CARTESIAN_POINT('Ctrl Pts',(-11.7989676549683,-72.004702016029,-20.1202732486577));
#27669=CARTESIAN_POINT('Ctrl Pts',(-11.7989014855416,-72.006459015246,-20.1240684980738));
#27670=CARTESIAN_POINT('Ctrl Pts',(-11.798830706444,-72.0082515438015,-20.1279403866504));
#27671=CARTESIAN_POINT('Ctrl Pts',(-11.7987541012368,-72.0101916225281,
-20.1321309858106));
#27672=CARTESIAN_POINT('Ctrl Pts',(-11.7986720719967,-72.0121730910341,
-20.1364108642537));
#27673=CARTESIAN_POINT('Ctrl Pts',(-11.7985851427786,-72.0141745494161,
-20.1407337886868));
#27674=CARTESIAN_POINT('Ctrl Pts',(-11.7984834837389,-72.0165151472244,
-20.1457892160414));
#27675=CARTESIAN_POINT('Ctrl Pts',(-11.7983750765891,-72.0188827135273,
-20.1509027131827));
#27676=CARTESIAN_POINT('Ctrl Pts',(-11.7982629359989,-72.0212129879397,
-20.1559354950726));
#27677=CARTESIAN_POINT('Ctrl Pts',(-11.7980988579961,-72.0246225185231,
-20.1632991873836));
#27678=CARTESIAN_POINT('Ctrl Pts',(-11.7979266789118,-72.0279487283432,
-20.1704825465795));
#27679=CARTESIAN_POINT('Ctrl Pts',(-11.797762638322,-72.0309524055999,-20.176969086863));
#27680=CARTESIAN_POINT('Ctrl Pts',(-11.7976578720253,-72.032870736562,-20.1811117859613));
#27681=CARTESIAN_POINT('Ctrl Pts',(-11.7975566186402,-72.0346567522059,
-20.184968628232));
#27682=CARTESIAN_POINT('Ctrl Pts',(-11.79746327233,-72.0362619878201,-20.1884350084057));
#27683=CARTESIAN_POINT('Ctrl Pts',(-11.7973769893237,-72.0377457588903,
-20.1916390954408));
#27684=CARTESIAN_POINT('Ctrl Pts',(-11.7972975249092,-72.0390746155401,
-20.1945085882328));
#27685=CARTESIAN_POINT('Ctrl Pts',(-11.7972272049842,-72.0402312692395,
-20.1970061974383));
#27686=CARTESIAN_POINT('Ctrl Pts',(-11.7971658232559,-72.0412409034669,
-20.1991863415397));
#27687=CARTESIAN_POINT('Ctrl Pts',(-11.7971114179676,-72.0421193686887,
-20.2010832179952));
#27688=CARTESIAN_POINT('Ctrl Pts',(-11.7970642228539,-72.0428738025906,
-20.2027122622304));
#27689=CARTESIAN_POINT('Ctrl Pts',(-11.7970188610415,-72.0435989303922,
-20.2042780259932));
#27690=CARTESIAN_POINT('Ctrl Pts',(-11.7969801733989,-72.0442093167846,
-20.2055960182921));
#27691=CARTESIAN_POINT('Ctrl Pts',(-11.7969468970578,-72.0447309306672,
-20.206722325243));
#27692=CARTESIAN_POINT('Ctrl Pts',(-11.7969151886715,-72.045227966516,-20.2077955615005));
#27693=CARTESIAN_POINT('Ctrl Pts',(-11.7968883962598,-72.0456443292891,
-20.208694601408));
#27694=CARTESIAN_POINT('Ctrl Pts',(-11.7968639638509,-72.0460222115476,
-20.2095105519188));
#27695=CARTESIAN_POINT('Ctrl Pts',(-11.7968490293866,-72.0462531944641,
-20.2100093068207));
#27696=CARTESIAN_POINT('Ctrl Pts',(-11.7968349480525,-72.0464701896551,
-20.210477858437));
#27697=CARTESIAN_POINT('Ctrl Pts',(-11.7968208397773,-72.0466869089798,
-20.2109458130836));
#27698=CARTESIAN_POINT('',(-11.73096720362,-72.9498142529578,-19.7928705604145));
#27699=CARTESIAN_POINT('Ctrl Pts',(-11.73096720362,-72.9498142529578,-19.7928705604145));
#27700=CARTESIAN_POINT('Ctrl Pts',(-11.7529184156725,-72.6487718049651,
-19.9322289779709));
#27701=CARTESIAN_POINT('Ctrl Pts',(-11.7748696277249,-72.3477293569724,
-20.0715873955272));
#27702=CARTESIAN_POINT('Ctrl Pts',(-11.7968208397773,-72.0466869089798,
-20.2109458130836));
#27703=CARTESIAN_POINT('',(-11.8,-72.5,-18.8097619285762));
#27704=CARTESIAN_POINT('Ctrl Pts',(-11.73096720362,-72.9498142529578,-19.7928705604145));
#27705=CARTESIAN_POINT('Ctrl Pts',(-11.7313015196475,-72.948750713357,-19.7904622157761));
#27706=CARTESIAN_POINT('Ctrl Pts',(-11.7316352664094,-72.9476850547636,
-19.7880498402146));
#27707=CARTESIAN_POINT('Ctrl Pts',(-11.7319930278409,-72.9465377567631,
-19.7854527057828));
#27708=CARTESIAN_POINT('Ctrl Pts',(-11.7323595526967,-72.9453623555119,
-19.7827919541218));
#27709=CARTESIAN_POINT('Ctrl Pts',(-11.7327512682097,-72.9441013208732,
-19.7799374057456));
#27710=CARTESIAN_POINT('Ctrl Pts',(-11.7331869939848,-72.9426906823876,
-19.7767444366006));
#27711=CARTESIAN_POINT('Ctrl Pts',(-11.7336348584884,-72.9412407454291,
-19.7734625156706));
#27712=CARTESIAN_POINT('Ctrl Pts',(-11.7341292070935,-72.9396328168219,
-19.7698231983777));
#27713=CARTESIAN_POINT('Ctrl Pts',(-11.7346827218845,-72.9378190122941,
-19.7657193035655));
#27714=CARTESIAN_POINT('Ctrl Pts',(-11.7352541156892,-72.9359466202874,
-19.7614828493476));
#27715=CARTESIAN_POINT('Ctrl Pts',(-11.7358885391894,-72.9338549102333,
-19.7567514881668));
#27716=CARTESIAN_POINT('Ctrl Pts',(-11.7365920277446,-72.9315128570745,
-19.7514573835512));
#27717=CARTESIAN_POINT('Ctrl Pts',(-11.737339030065,-72.9290259379468,-19.7458358160034));
#27718=CARTESIAN_POINT('Ctrl Pts',(-11.7381638939142,-72.9262567549538,
-19.7395797634214));
#27719=CARTESIAN_POINT('Ctrl Pts',(-11.7390652426951,-72.9231917145537,
-19.7326623884211));
#27720=CARTESIAN_POINT('Ctrl Pts',(-11.7400142162781,-72.9199647258095,
-19.7253795182624));
#27721=CARTESIAN_POINT('Ctrl Pts',(-11.7410478975251,-72.9164098863763,
-19.7173638520341));
#27722=CARTESIAN_POINT('Ctrl Pts',(-11.742156091357,-72.9125358265191,-19.7086402756966));
#27723=CARTESIAN_POINT('Ctrl Pts',(-11.743343246297,-72.9083857318654,-19.6992951264596));
#27724=CARTESIAN_POINT('Ctrl Pts',(-11.7446157812005,-72.9038694321553,
-19.6891379476566));
#27725=CARTESIAN_POINT('Ctrl Pts',(-11.7459531151839,-72.8990232934177,
-19.678257641115));
#27726=CARTESIAN_POINT('Ctrl Pts',(-11.7474361285517,-72.8936492517657,
-19.6661921135459));
#27727=CARTESIAN_POINT('Ctrl Pts',(-11.7489985853597,-72.8878697945666,
-19.6532379065394));
#27728=CARTESIAN_POINT('Ctrl Pts',(-11.7506057804669,-72.881762844808,-19.6395787832203));
#27729=CARTESIAN_POINT('Ctrl Pts',(-11.7525799686944,-72.8742614106234,
-19.6228006830806));
#27730=CARTESIAN_POINT('Ctrl Pts',(-11.7546209594929,-72.8662663671094,
-19.604960507791));
#27731=CARTESIAN_POINT('Ctrl Pts',(-11.7566625088008,-72.8579585666724,
-19.586474830845));
#27732=CARTESIAN_POINT('Ctrl Pts',(-11.7587486675852,-72.8494692341864,
-19.5675852271509));
#27733=CARTESIAN_POINT('Ctrl Pts',(-11.7608345555821,-72.8406557779562,
-19.5480271717187));
#27734=CARTESIAN_POINT('Ctrl Pts',(-11.7628608882688,-72.8317197937618,
-19.5282555924746));
#27735=CARTESIAN_POINT('Ctrl Pts',(-11.7644778516186,-72.8245890994631,
-19.5124783614135));
#27736=CARTESIAN_POINT('Ctrl Pts',(-11.7660570732259,-72.8173810768957,
-19.4965664860538));
#27737=CARTESIAN_POINT('Ctrl Pts',(-11.7675779301993,-72.8101854587048,
-19.4807189446334));
#27738=CARTESIAN_POINT('Ctrl Pts',(-11.7689362640305,-72.8037587849308,
-19.4665649169842));
#27739=CARTESIAN_POINT('Ctrl Pts',(-11.7702481416314,-72.797342265795,-19.4524626966761));
#27740=CARTESIAN_POINT('Ctrl Pts',(-11.7715056463165,-72.7909830456549,
-19.4385150048574));
#27741=CARTESIAN_POINT('Ctrl Pts',(-11.7726775448823,-72.7850567369498,
-19.4255168186616));
#27742=CARTESIAN_POINT('Ctrl Pts',(-11.7738022936455,-72.7791803623659,
-19.4126531659137));
#27743=CARTESIAN_POINT('Ctrl Pts',(-11.7748785745449,-72.7733737191987,
-19.3999657098098));
#27744=CARTESIAN_POINT('Ctrl Pts',(-11.7759007008184,-72.7678592456579,
-19.3879166413602));
#27745=CARTESIAN_POINT('Ctrl Pts',(-11.7768791728643,-72.7624077892709,
-19.3760267312504));
#27746=CARTESIAN_POINT('Ctrl Pts',(-11.7778167135231,-72.7570170446327,
-19.3642888201112));
#27747=CARTESIAN_POINT('Ctrl Pts',(-11.7787167543063,-72.7518419197138,
-19.3530204034994));
#27748=CARTESIAN_POINT('Ctrl Pts',(-11.7795791232979,-72.7467228466605,
-19.3418922673075));
#27749=CARTESIAN_POINT('Ctrl Pts',(-11.7804091012626,-72.7416379376232,
-19.3308543416171));
#27750=CARTESIAN_POINT('Ctrl Pts',(-11.7812615549807,-72.7364153295549,
-19.3195175095628));
#27751=CARTESIAN_POINT('Ctrl Pts',(-11.7820798790364,-72.7312290756134,
-19.3082765101024));
#27752=CARTESIAN_POINT('Ctrl Pts',(-11.78287228708,-72.7260304851342,-19.2970224013524));
#27753=CARTESIAN_POINT('Ctrl Pts',(-11.7836281622423,-72.7210715685085,
-19.2862871477848));
#27754=CARTESIAN_POINT('Ctrl Pts',(-11.7843609633582,-72.7160978816426,
-19.2755321855914));
#27755=CARTESIAN_POINT('Ctrl Pts',(-11.7850752081796,-72.7110725611027,
-19.2646751402817));
#27756=CARTESIAN_POINT('Ctrl Pts',(-11.7858149458742,-72.7058678764904,
-19.2534305845943));
#27757=CARTESIAN_POINT('Ctrl Pts',(-11.7865346992853,-72.7006078834654,
-19.2420767205995));
#27758=CARTESIAN_POINT('Ctrl Pts',(-11.787234971241,-72.6952745255222,-19.2305723846674));
#27759=CARTESIAN_POINT('Ctrl Pts',(-11.787983905607,-72.6895705486344,-19.2182686040163));
#27760=CARTESIAN_POINT('Ctrl Pts',(-11.7887104701913,-72.6837826658412,
-19.2057927574211));
#27761=CARTESIAN_POINT('Ctrl Pts',(-11.7894114938235,-72.6779140299877,
-19.1931496137544));
#27762=CARTESIAN_POINT('Ctrl Pts',(-11.7901552177242,-72.67168792783,-19.1797363596303));
#27763=CARTESIAN_POINT('Ctrl Pts',(-11.790870062336,-72.6653710751155,-19.1661351349512));
#27764=CARTESIAN_POINT('Ctrl Pts',(-11.7915498844441,-72.6589935288453,
-19.1524086643696));
#27765=CARTESIAN_POINT('Ctrl Pts',(-11.7922885192423,-72.6520642490451,
-19.1374946909855));
#27766=CARTESIAN_POINT('Ctrl Pts',(-11.7929856244291,-72.6450635375576,
-19.1224333550758));
#27767=CARTESIAN_POINT('Ctrl Pts',(-11.7936332018617,-72.6380574456386,
-19.1073643771971));
#27768=CARTESIAN_POINT('Ctrl Pts',(-11.7943843329216,-72.6299310147553,
-19.0898857302383));
#27769=CARTESIAN_POINT('Ctrl Pts',(-11.7950684833757,-72.6217977656785,
-19.0723977162336));
#27770=CARTESIAN_POINT('Ctrl Pts',(-11.7956775773033,-72.6137918483554,
-19.0551850309453));
#27771=CARTESIAN_POINT('Ctrl Pts',(-11.7964581312637,-72.6035322640937,
-19.0331269721424));
#27772=CARTESIAN_POINT('Ctrl Pts',(-11.7971144717794,-72.5934842779128,
-19.0115263327855));
#27773=CARTESIAN_POINT('Ctrl Pts',(-11.7976485571115,-72.5839571282364,
-18.991040307301));
#27774=CARTESIAN_POINT('Ctrl Pts',(-11.7980302737727,-72.5771479695768,
-18.9763987195685));
#27775=CARTESIAN_POINT('Ctrl Pts',(-11.798350091132,-72.5706057723494,-18.9623284432994));
#27776=CARTESIAN_POINT('Ctrl Pts',(-11.7986154805682,-72.5644332321203,
-18.9490480921655));
#27777=CARTESIAN_POINT('Ctrl Pts',(-11.7988537013714,-72.5588925914945,
-18.9371272864217));
#27778=CARTESIAN_POINT('Ctrl Pts',(-11.7990482195448,-72.5536501203106,
-18.9258436471241));
#27779=CARTESIAN_POINT('Ctrl Pts',(-11.7992071495588,-72.548763948896,-18.9153211964204));
#27780=CARTESIAN_POINT('Ctrl Pts',(-11.7993555434031,-72.5442017032746,
-18.9054963252532));
#27781=CARTESIAN_POINT('Ctrl Pts',(-11.7994730024161,-72.5399502820446,
-18.8963354982137));
#27782=CARTESIAN_POINT('Ctrl Pts',(-11.7995670103527,-72.5360386107081,
-18.8879006581774));
#27783=CARTESIAN_POINT('Ctrl Pts',(-11.799656382681,-72.5323198270885,-18.8798817470105));
#27784=CARTESIAN_POINT('Ctrl Pts',(-11.7997246147799,-72.528908256622,-18.8725193061859));
#27785=CARTESIAN_POINT('Ctrl Pts',(-11.7997779466319,-72.5258091223535,
-18.8658247654831));
#27786=CARTESIAN_POINT('Ctrl Pts',(-11.7998291813466,-72.5228318535359,
-18.8593934703034));
#27787=CARTESIAN_POINT('Ctrl Pts',(-11.7998666928443,-72.5201430448025,
-18.853578828993));
#27788=CARTESIAN_POINT('Ctrl Pts',(-11.7998952486479,-72.5177269028185,
-18.8483473576186));
#27789=CARTESIAN_POINT('Ctrl Pts',(-11.7999224505255,-72.5154253181936,
-18.8433639277702));
#27790=CARTESIAN_POINT('Ctrl Pts',(-11.7999415314462,-72.5133711920832,
-18.8389097591737));
#27791=CARTESIAN_POINT('Ctrl Pts',(-11.7999556780829,-72.5115309924458,
-18.8349133524625));
#27792=CARTESIAN_POINT('Ctrl Pts',(-11.7999695052011,-72.5097323559027,
-18.8310072093431));
#27793=CARTESIAN_POINT('Ctrl Pts',(-11.7999786158405,-72.5081381840189,
-18.8275385858994));
#27794=CARTESIAN_POINT('Ctrl Pts',(-11.7999850514837,-72.5066966652379,
-18.8243967636039));
#27795=CARTESIAN_POINT('Ctrl Pts',(-11.7999912849267,-72.5053004372806,
-18.8213536536676));
#27796=CARTESIAN_POINT('Ctrl Pts',(-11.7999950012486,-72.5040474593205,
-18.8186172172743));
#27797=CARTESIAN_POINT('Ctrl Pts',(-11.7999972537808,-72.5028703048568,
-18.8160431764752));
#27798=CARTESIAN_POINT('Ctrl Pts',(-11.7999991536502,-72.5018774490286,
-18.8138721347909));
#27799=CARTESIAN_POINT('Ctrl Pts',(-11.8,-72.500938234387,-18.8118159787353));
#27800=CARTESIAN_POINT('Ctrl Pts',(-11.8,-72.5,-18.8097619285762));
#27801=CARTESIAN_POINT('',(-11.8,-72.2245134174903,-19.4048809642881));
#27802=CARTESIAN_POINT('Ctrl Pts',(-11.73096720362,-72.9498142529578,-19.7928705604145));
#27803=CARTESIAN_POINT('Ctrl Pts',(-11.6459067968618,-73.2204118420674,
-20.405628423336));
#27804=CARTESIAN_POINT('Ctrl Pts',(-11.3040150424387,-73.7466604863582,
-21.7070034589623));
#27805=CARTESIAN_POINT('Ctrl Pts',(-10.6578917243185,-74.000000000005,-22.9273203194824));
#27806=CARTESIAN_POINT('Ctrl Pts',(-10.299999999979,-74.,-23.4706975310694));
#27807=CARTESIAN_POINT('Ctrl Pts',(-11.7529184156725,-72.6487718049651,
-19.9322289779709));
#27808=CARTESIAN_POINT('Ctrl Pts',(-11.6900562551077,-72.9237214947494,
-20.5448956110034));
#27809=CARTESIAN_POINT('Ctrl Pts',(-11.3929734933996,-73.4750028661316,
-21.8418300905598));
#27810=CARTESIAN_POINT('Ctrl Pts',(-10.7749647057687,-73.7841592833289,
-23.0483683735484));
#27811=CARTESIAN_POINT('Ctrl Pts',(-10.4245617157746,-73.8157835059031,
-23.5830861153787));
#27812=CARTESIAN_POINT('Ctrl Pts',(-11.7748696277249,-72.3477293569724,
-20.0715873955272));
#27813=CARTESIAN_POINT('Ctrl Pts',(-11.7342057133535,-72.6270311474313,
-20.6841627986708));
#27814=CARTESIAN_POINT('Ctrl Pts',(-11.4819319443604,-73.203345245905,-21.9766567221572));
#27815=CARTESIAN_POINT('Ctrl Pts',(-10.8920376872188,-73.5683185666529,
-23.1694164276145));
#27816=CARTESIAN_POINT('Ctrl Pts',(-10.5491234315702,-73.6315670118062,
-23.6954746996879));
#27817=CARTESIAN_POINT('Ctrl Pts',(-11.7968208397773,-72.0466869089798,
-20.2109458130836));
#27818=CARTESIAN_POINT('Ctrl Pts',(-11.7783551715994,-72.3303408001132,
-20.8234299863382));
#27819=CARTESIAN_POINT('Ctrl Pts',(-11.5708903953213,-72.9316876256785,
-22.1114833537547));
#27820=CARTESIAN_POINT('Ctrl Pts',(-11.009110668669,-73.3524778499768,-23.2904644816805));
#27821=CARTESIAN_POINT('Ctrl Pts',(-10.6736851473658,-73.4473505177094,
-23.8078632839972));
#27822=CARTESIAN_POINT('',(-10.6736851473658,-73.4473505177094,-23.8078632839972));
#27823=CARTESIAN_POINT('Ctrl Pts',(-11.7968208397773,-72.0466869089798,
-20.2109458130836));
#27824=CARTESIAN_POINT('Ctrl Pts',(-11.7783551715994,-72.3303408001132,
-20.8234299863382));
#27825=CARTESIAN_POINT('Ctrl Pts',(-11.5708903953213,-72.9316876256785,
-22.1114833537547));
#27826=CARTESIAN_POINT('Ctrl Pts',(-11.009110668669,-73.3524778499768,-23.2904644816805));
#27827=CARTESIAN_POINT('Ctrl Pts',(-10.6736851473658,-73.4473505177094,
-23.8078632839972));
#27828=CARTESIAN_POINT('',(-10.2999999999876,-74.,-23.4706975310751));
#27829=CARTESIAN_POINT('',(-10.6736851473658,-73.4473505177094,-23.8078632839972));
#27830=CARTESIAN_POINT('Ctrl Pts',(-10.299999999979,-74.,-23.4706975310694));
#27831=CARTESIAN_POINT('Ctrl Pts',(-10.6578917243185,-74.000000000005,-22.9273203194824));
#27832=CARTESIAN_POINT('Ctrl Pts',(-11.3040150424387,-73.7466604863582,
-21.7070034589623));
#27833=CARTESIAN_POINT('Ctrl Pts',(-11.6459067968618,-73.2204118420674,
-20.405628423336));
#27834=CARTESIAN_POINT('Ctrl Pts',(-11.73096720362,-72.9498142529578,-19.7928705604145));
#27835=CARTESIAN_POINT('Origin',(-4.79999999999999,-73.75,-20.));
#27836=CARTESIAN_POINT('',(-9.13012701892219,-73.5,-25.5));
#27837=CARTESIAN_POINT('',(-8.82083223185632,-74.,-25.1071428571429));
#27838=CARTESIAN_POINT('',(-9.13012701892219,-73.5,-25.5));
#27839=CARTESIAN_POINT('',(-9.90714285714286,-74.,-24.0208322318563));
#27840=CARTESIAN_POINT('Origin',(-4.79999999999999,-74.,-20.));
#27841=CARTESIAN_POINT('',(-10.3,-73.5,-24.3301270189222));
#27842=CARTESIAN_POINT('',(-9.90714285714286,-74.,-24.0208322318563));
#27843=CARTESIAN_POINT('Origin',(-4.79999999999999,-73.5,-20.));
#27844=CARTESIAN_POINT('Ctrl Pts',(-10.299999999979,-74.,-23.4706975310694));
#27845=CARTESIAN_POINT('Ctrl Pts',(-10.1730966676381,-74.,-23.6633713879345));
#27846=CARTESIAN_POINT('Ctrl Pts',(-10.0446625272125,-74.,-23.8461587910824));
#27847=CARTESIAN_POINT('Ctrl Pts',(-9.90714285714286,-74.,-24.0208322318563));
#27848=CARTESIAN_POINT('Ctrl Pts',(-10.4245617157746,-73.8157835059031,
-23.5830861153787));
#27849=CARTESIAN_POINT('Ctrl Pts',(-10.3003137824799,-73.8269970069562,
-23.7726894470159));
#27850=CARTESIAN_POINT('Ctrl Pts',(-10.1728443653613,-73.8333333333333,
-23.9527761154313));
#27851=CARTESIAN_POINT('Ctrl Pts',(-10.0380952380952,-73.8333333333333,
-24.1239304942116));
#27852=CARTESIAN_POINT('Ctrl Pts',(-10.5491234315702,-73.6315670118063,
-23.6954746996879));
#27853=CARTESIAN_POINT('Ctrl Pts',(-10.4275308973216,-73.6539940139125,
-23.8820075060973));
#27854=CARTESIAN_POINT('Ctrl Pts',(-10.3010262035101,-73.6666666666667,
-24.0593934397802));
#27855=CARTESIAN_POINT('Ctrl Pts',(-10.1690476190476,-73.6666666666667,
-24.2270287565669));
#27856=CARTESIAN_POINT('Ctrl Pts',(-10.6736851473658,-73.4473505177094,
-23.8078632839972));
#27857=CARTESIAN_POINT('Ctrl Pts',(-10.5547480121633,-73.4809910208687,
-23.9913255651787));
#27858=CARTESIAN_POINT('Ctrl Pts',(-10.4292080416588,-73.5,-24.1660107641291));
#27859=CARTESIAN_POINT('Ctrl Pts',(-10.3,-73.5,-24.3301270189222));
#27860=CARTESIAN_POINT('Ctrl Pts',(-9.90714285714286,-74.,-24.0208322318563));
#27861=CARTESIAN_POINT('Ctrl Pts',(-10.0446625272125,-74.,-23.8461587910824));
#27862=CARTESIAN_POINT('Ctrl Pts',(-10.1730966676381,-74.,-23.6633713879345));
#27863=CARTESIAN_POINT('Ctrl Pts',(-10.299999999979,-74.,-23.4706975310694));
#27864=CARTESIAN_POINT('Ctrl Pts',(-10.6736851473658,-73.4473505177094,
-23.8078632839972));
#27865=CARTESIAN_POINT('Ctrl Pts',(-10.5547480121633,-73.4809910208687,
-23.9913255651787));
#27866=CARTESIAN_POINT('Ctrl Pts',(-10.4292080416588,-73.5,-24.1660107641291));
#27867=CARTESIAN_POINT('Ctrl Pts',(-10.3,-73.5,-24.3301270189222));
#27868=CARTESIAN_POINT('Ctrl Pts',(-8.27069753274498,-74.,-25.4999999988754));
#27869=CARTESIAN_POINT('Ctrl Pts',(-7.86775357562108,-74.000000000199,-25.7653963103419));
#27870=CARTESIAN_POINT('Ctrl Pts',(-7.41892233716379,-73.9255855959792,
-26.0143834333207));
#27871=CARTESIAN_POINT('Ctrl Pts',(-6.64131213535275,-73.7333039309982,
-26.3751847566866));
#27872=CARTESIAN_POINT('Ctrl Pts',(-6.23069752441905,-73.6032053694849,
-26.5355631282739));
#27873=CARTESIAN_POINT('Ctrl Pts',(-5.3994360061265,-73.2960267407261,-26.7866346555581));
#27874=CARTESIAN_POINT('Ctrl Pts',(-4.97871567190643,-73.1202058398724,
-26.8774059891363));
#27875=CARTESIAN_POINT('Ctrl Pts',(-4.59286786251854,-72.9498130615488,
-26.9309675781303));
#27876=CARTESIAN_POINT('Ctrl Pts',(-8.38308611702755,-73.8157835060006,
-25.6245617146941));
#27877=CARTESIAN_POINT('Ctrl Pts',(-7.98659795770256,-73.792224809411,-25.8845123595968));
#27878=CARTESIAN_POINT('Ctrl Pts',(-7.54321375147387,-73.6962979999651,
-26.1239924943787));
#27879=CARTESIAN_POINT('Ctrl Pts',(-6.77293317326111,-73.4735100646501,
-26.4648563557158));
#27880=CARTESIAN_POINT('Ctrl Pts',(-6.36525357393195,-73.3302738061139,
-26.6131752565609));
#27881=CARTESIAN_POINT('Ctrl Pts',(-5.53781831770394,-73.0038693973692,
-26.8373085713286));
#27882=CARTESIAN_POINT('Ctrl Pts',(-5.11803369719418,-72.8218328925055,
-26.9133546198602));
#27883=CARTESIAN_POINT('Ctrl Pts',(-4.73222628093364,-72.6487705946061,
-26.9529186924327));
#27884=CARTESIAN_POINT('Ctrl Pts',(-8.49547470131012,-73.6315670120013,
-25.7491234305128));
#27885=CARTESIAN_POINT('Ctrl Pts',(-8.10533935942276,-73.5847724307058,
-26.0033054887914));
#27886=CARTESIAN_POINT('Ctrl Pts',(-7.66749386372855,-73.4670506442876,
-26.2335668887596));
#27887=CARTESIAN_POINT('Ctrl Pts',(-6.90453529773527,-73.2137792063844,
-26.5544816958254));
#27888=CARTESIAN_POINT('Ctrl Pts',(-6.49978151201769,-73.0574412945255,
-26.6907208978012));
#27889=CARTESIAN_POINT('Ctrl Pts',(-5.6762040020745,-72.7117043334441,-26.8879935435987));
#27890=CARTESIAN_POINT('Ctrl Pts',(-5.25729945114597,-72.523672254769,-26.9492448165541));
#27891=CARTESIAN_POINT('Ctrl Pts',(-4.87158469934875,-72.3477281276634,
-26.9748698067351));
#27892=CARTESIAN_POINT('Ctrl Pts',(-8.60786328559269,-73.4473505180019,
-25.8736851463315));
#27893=CARTESIAN_POINT('Ctrl Pts',(-8.22418374150425,-73.3769972399179,
-26.1224215380463));
#27894=CARTESIAN_POINT('Ctrl Pts',(-7.79178527803863,-73.2377630482735,
-26.3431759498177));
#27895=CARTESIAN_POINT('Ctrl Pts',(-7.03615633564364,-72.9539853400363,
-26.6441532948547));
#27896=CARTESIAN_POINT('Ctrl Pts',(-6.63433756153059,-72.7845097311546,
-26.7683330260882));
#27897=CARTESIAN_POINT('Ctrl Pts',(-5.81458631365194,-72.4195469900871,
-26.9386674593692));
#27898=CARTESIAN_POINT('Ctrl Pts',(-5.39661747643372,-72.2252993074021,
-26.985193447278));
#27899=CARTESIAN_POINT('Ctrl Pts',(-5.01094311776385,-72.0466856607207,
-26.9968209210375));
#27900=CARTESIAN_POINT('',(-8.27069753304877,-74.,-25.4999999993376));
#27901=CARTESIAN_POINT('Ctrl Pts',(-4.59286786251854,-72.9498130615488,
-26.9309675781303));
#27902=CARTESIAN_POINT('Ctrl Pts',(-4.97871567190643,-73.1202058398724,
-26.8774059891363));
#27903=CARTESIAN_POINT('Ctrl Pts',(-5.3994360061265,-73.2960267407261,-26.7866346555581));
#27904=CARTESIAN_POINT('Ctrl Pts',(-6.23069752441905,-73.6032053694849,
-26.5355631282739));
#27905=CARTESIAN_POINT('Ctrl Pts',(-6.64131213535275,-73.7333039309982,
-26.3751847566866));
#27906=CARTESIAN_POINT('Ctrl Pts',(-7.41892233716379,-73.9255855959792,
-26.0143834333207));
#27907=CARTESIAN_POINT('Ctrl Pts',(-7.86775357562108,-74.000000000199,-25.7653963103419));
#27908=CARTESIAN_POINT('Ctrl Pts',(-8.27069753274498,-74.,-25.4999999988754));
#27909=CARTESIAN_POINT('',(-8.60786328559223,-73.4473505180018,-25.8736851463318));
#27910=CARTESIAN_POINT('',(-8.27069753304877,-74.,-25.4999999993376));
#27911=CARTESIAN_POINT('Ctrl Pts',(-8.60786328559269,-73.4473505180019,
-25.8736851463315));
#27912=CARTESIAN_POINT('Ctrl Pts',(-8.22418374150425,-73.3769972399179,
-26.1224215380463));
#27913=CARTESIAN_POINT('Ctrl Pts',(-7.79178527803863,-73.2377630482735,
-26.3431759498177));
#27914=CARTESIAN_POINT('Ctrl Pts',(-7.03615633564364,-72.9539853400363,
-26.6441532948547));
#27915=CARTESIAN_POINT('Ctrl Pts',(-6.63433756153059,-72.7845097311546,
-26.7683330260882));
#27916=CARTESIAN_POINT('Ctrl Pts',(-5.81458631365194,-72.4195469900871,
-26.9386674593692));
#27917=CARTESIAN_POINT('Ctrl Pts',(-5.39661747643372,-72.2252993074021,
-26.985193447278));
#27918=CARTESIAN_POINT('Ctrl Pts',(-5.01094311776385,-72.0466856607207,
-26.9968209210375));
#27919=CARTESIAN_POINT('Ctrl Pts',(-8.82083223185632,-74.,-25.1071428571429));
#27920=CARTESIAN_POINT('Ctrl Pts',(-8.6524411521674,-74.,-25.2397164505804));
#27921=CARTESIAN_POINT('Ctrl Pts',(-8.46780983228827,-74.,-25.3701733162485));
#27922=CARTESIAN_POINT('Ctrl Pts',(-8.2706975327445,-74.,-25.4999999988757));
#27923=CARTESIAN_POINT('Ctrl Pts',(-8.92393049421161,-73.8333333333333,
-25.2380952380952));
#27924=CARTESIAN_POINT('Ctrl Pts',(-8.75893190880213,-73.8333333333333,
-25.3679979349617));
#27925=CARTESIAN_POINT('Ctrl Pts',(-8.57705715860084,-73.8272553216869,
-25.4974516009823));
#27926=CARTESIAN_POINT('Ctrl Pts',(-8.38308611702708,-73.8157835060006,
-25.6245617146944));
#27927=CARTESIAN_POINT('Ctrl Pts',(-9.0270287565669,-73.6666666666667,-25.3690476190476));
#27928=CARTESIAN_POINT('Ctrl Pts',(-8.86542266543687,-73.6666666666667,
-25.496279419343));
#27929=CARTESIAN_POINT('Ctrl Pts',(-8.68630448491342,-73.6545106433737,
-25.6247298857161));
#27930=CARTESIAN_POINT('Ctrl Pts',(-8.49547470130966,-73.6315670120012,
-25.7491234305131));
#27931=CARTESIAN_POINT('Ctrl Pts',(-9.13012701892219,-73.5,-25.5));
#27932=CARTESIAN_POINT('Ctrl Pts',(-8.97191342207161,-73.5,-25.6245609037243));
#27933=CARTESIAN_POINT('Ctrl Pts',(-8.79555181122599,-73.4817659650606,
-25.7520081704499));
#27934=CARTESIAN_POINT('Ctrl Pts',(-8.60786328559223,-73.4473505180018,
-25.8736851463318));
#27935=CARTESIAN_POINT('Ctrl Pts',(-8.2706975327445,-74.,-25.4999999988757));
#27936=CARTESIAN_POINT('Ctrl Pts',(-8.46780983228827,-74.,-25.3701733162485));
#27937=CARTESIAN_POINT('Ctrl Pts',(-8.6524411521674,-74.,-25.2397164505804));
#27938=CARTESIAN_POINT('Ctrl Pts',(-8.82083223185632,-74.,-25.1071428571429));
#27939=CARTESIAN_POINT('Ctrl Pts',(-9.13012701892219,-73.5,-25.5));
#27940=CARTESIAN_POINT('Ctrl Pts',(-8.97191342207161,-73.5,-25.6245609037243));
#27941=CARTESIAN_POINT('Ctrl Pts',(-8.79555181122599,-73.4817659650606,
-25.7520081704499));
#27942=CARTESIAN_POINT('Ctrl Pts',(-8.60786328559223,-73.4473505180018,
-25.8736851463318));
#27943=CARTESIAN_POINT('Origin',(5.2,-72.5,-25.5));
#27944=CARTESIAN_POINT('',(34.9928690003034,-72.9498135639887,-26.9309674201923));
#27945=CARTESIAN_POINT('Ctrl Pts',(34.9928690003034,-72.9498135639887,-26.9309674201923));
#27946=CARTESIAN_POINT('Ctrl Pts',(34.9904606339408,-72.948750014595,-26.9313017387355));
#27947=CARTESIAN_POINT('Ctrl Pts',(34.98804823666,-72.9476843461928,-26.9316354879942));
#27948=CARTESIAN_POINT('Ctrl Pts',(34.9854510809667,-72.9465370382985,-26.9319932518792));
#27949=CARTESIAN_POINT('Ctrl Pts',(34.9827903074055,-72.9453616268591,-26.9323597792649));
#27950=CARTESIAN_POINT('Ctrl Pts',(34.9799357375926,-72.944100581936,-26.9327514972644));
#27951=CARTESIAN_POINT('Ctrl Pts',(34.9767427478805,-72.9426899331038,-26.9331872254275));
#27952=CARTESIAN_POINT('Ctrl Pts',(34.9734608056225,-72.9412399854274,-26.9336350924113));
#27953=CARTESIAN_POINT('Ctrl Pts',(34.9698214678795,-72.9396320460192,-26.9341294433976));
#27954=CARTESIAN_POINT('Ctrl Pts',(34.9657175538563,-72.9378182307483,-26.9346829603869));
#27955=CARTESIAN_POINT('Ctrl Pts',(34.9614810794814,-72.9359458275077,-26.9352543565048));
#27956=CARTESIAN_POINT('Ctrl Pts',(34.9567496993881,-72.9338541062487,-26.9358887821325));
#27957=CARTESIAN_POINT('Ctrl Pts',(34.9514555774257,-72.9315120421697,-26.9365922725194));
#27958=CARTESIAN_POINT('Ctrl Pts',(34.9458339906315,-72.9290251110807,-26.9373392768946));
#27959=CARTESIAN_POINT('Ctrl Pts',(34.9395779203818,-72.9262559163651,-26.9381641424873));
#27960=CARTESIAN_POINT('Ctrl Pts',(34.9326605296007,-72.9231908648904,-26.9390654925587));
#27961=CARTESIAN_POINT('Ctrl Pts',(34.9253776414208,-72.9199638638632,-26.9400144676838));
#27962=CARTESIAN_POINT('Ctrl Pts',(34.9173619589799,-72.9164090127403,-26.9410481500021));
#27963=CARTESIAN_POINT('Ctrl Pts',(34.9086383685528,-72.9125349423719,-26.9421563442714));
#27964=CARTESIAN_POINT('Ctrl Pts',(34.8992932010295,-72.9083848350403,-26.9433435000854));
#27965=CARTESIAN_POINT('Ctrl Pts',(34.8891360058222,-72.9038685237575,-26.9446160351915));
#27966=CARTESIAN_POINT('Ctrl Pts',(34.8782556851746,-72.8990223753931,-26.9459533685205));
#27967=CARTESIAN_POINT('Ctrl Pts',(34.8661901327592,-72.8936483189661,-26.9474363822937));
#27968=CARTESIAN_POINT('Ctrl Pts',(34.8532359023791,-72.8878688487729,-26.9489988385702));
#27969=CARTESIAN_POINT('Ctrl Pts',(34.8395767580721,-72.8817618891628,-26.9506060319683));
#27970=CARTESIAN_POINT('Ctrl Pts',(34.8227985438473,-72.8742604033963,-26.9525802284866));
#27971=CARTESIAN_POINT('Ctrl Pts',(34.8049582468976,-72.8662653078647,-26.9546212264818));
#27972=CARTESIAN_POINT('Ctrl Pts',(34.7864724488064,-72.8579574601953,-26.9566627807048));
#27973=CARTESIAN_POINT('Ctrl Pts',(34.7675828912716,-72.8494681558239,-26.9587489257425));
#27974=CARTESIAN_POINT('Ctrl Pts',(34.7480248947017,-72.8406547386309,-26.9608347976192));
#27975=CARTESIAN_POINT('Ctrl Pts',(34.7282533823277,-72.8317188036679,-26.9628611127832));
#27976=CARTESIAN_POINT('Ctrl Pts',(34.7124762273523,-72.8245881589253,-26.9644780598212));
#27977=CARTESIAN_POINT('Ctrl Pts',(34.696564433511,-72.8173801925988,-26.9660572643433));
#27978=CARTESIAN_POINT('Ctrl Pts',(34.6807169754739,-72.8101846360259,-26.9675781040795));
#27979=CARTESIAN_POINT('Ctrl Pts',(34.6665630018486,-72.8037580080004,-26.9689364244778));
#27980=CARTESIAN_POINT('Ctrl Pts',(34.6524608371956,-72.7973415389273,-26.97024828839));
#27981=CARTESIAN_POINT('Ctrl Pts',(34.6385132007751,-72.7909823722005,-26.9715057794887));
#27982=CARTESIAN_POINT('Ctrl Pts',(34.6255150592532,-72.7850561101023,-26.9726776660199));
#27983=CARTESIAN_POINT('Ctrl Pts',(34.6126514510974,-72.7791797850873,-26.9738024027868));
#27984=CARTESIAN_POINT('Ctrl Pts',(34.5999640381744,-72.7733731934708,-26.9748786719902));
#27985=CARTESIAN_POINT('Ctrl Pts',(34.5879150073292,-72.7678587673291,-26.9759007874449));
#27986=CARTESIAN_POINT('Ctrl Pts',(34.5760251336394,-72.7624073601635,-26.9768792489179));
#27987=CARTESIAN_POINT('Ctrl Pts',(34.5642872567015,-72.7570166655066,-26.9778167794594));
#27988=CARTESIAN_POINT('Ctrl Pts',(34.5530188709448,-72.7518415876615,-26.9787168106879));
#27989=CARTESIAN_POINT('Ctrl Pts',(34.5418907636116,-72.7467225624016,-26.9795791705311));
#27990=CARTESIAN_POINT('Ctrl Pts',(34.5308528639428,-72.7416377007136,-26.9804091399319));
#27991=CARTESIAN_POINT('Ctrl Pts',(34.5195158985983,-72.7364150675617,-26.9812615968862));
#27992=CARTESIAN_POINT('Ctrl Pts',(34.5082747656363,-72.7312287891322,-26.9820799238305));
#27993=CARTESIAN_POINT('Ctrl Pts',(34.4970205175406,-72.7260301710798,-26.9828723349505));
#27994=CARTESIAN_POINT('Ctrl Pts',(34.4862852692864,-72.7210712920061,-26.9836282033142));
#27995=CARTESIAN_POINT('Ctrl Pts',(34.4755303076514,-72.7160976402511,-26.9843609983882));
#27996=CARTESIAN_POINT('Ctrl Pts',(34.4646732598926,-72.7110723522028,-26.9850752378703));
#27997=CARTESIAN_POINT('Ctrl Pts',(34.4534286993624,-72.7058677001745,-26.9858149701869));
#27998=CARTESIAN_POINT('Ctrl Pts',(34.4420748272551,-72.7006077369017,-26.9865347189658));
#27999=CARTESIAN_POINT('Ctrl Pts',(34.430570481744,-72.6952744058455,-26.9872349869545));
#28000=CARTESIAN_POINT('Ctrl Pts',(34.4182666858938,-72.6895704554162,-26.9879839173797));
#28001=CARTESIAN_POINT('Ctrl Pts',(34.4057908222855,-72.6837825957362,-26.988710478766));
#28002=CARTESIAN_POINT('Ctrl Pts',(34.3931476618623,-72.677913979816,-26.9894114998166));
#28003=CARTESIAN_POINT('Ctrl Pts',(34.3797343823661,-72.6716878952801,-26.9901552213997));
#28004=CARTESIAN_POINT('Ctrl Pts',(34.3661331323945,-72.6653710565065,-26.9908700643537));
#28005=CARTESIAN_POINT('Ctrl Pts',(34.3524066390149,-72.6589935209781,-26.9915498852828));
#28006=CARTESIAN_POINT('Ctrl Pts',(34.3374926243335,-72.6520642451703,-26.9922885196183));
#28007=CARTESIAN_POINT('Ctrl Pts',(34.3224312497526,-72.6450635337418,-26.9929856248129));
#28008=CARTESIAN_POINT('Ctrl Pts',(34.3073622391497,-72.6380574390556,-26.9936332024702));
#28009=CARTESIAN_POINT('Ctrl Pts',(34.2898834604621,-72.6299309613649,-26.9943843378204));
#28010=CARTESIAN_POINT('Ctrl Pts',(34.2723953226409,-72.6217976616031,-26.995068492125));
#28011=CARTESIAN_POINT('Ctrl Pts',(34.2551825307308,-72.6137916939583,-26.9956775890499));
#28012=CARTESIAN_POINT('Ctrl Pts',(34.2331249689417,-72.6035323399309,-26.9964581244288));
#28013=CARTESIAN_POINT('Ctrl Pts',(34.2115248288828,-72.5934845725505,-26.9971144521715));
#28014=CARTESIAN_POINT('Ctrl Pts',(34.1910392653848,-72.5839576125602,-26.9976485299606));
#28015=CARTESIAN_POINT('Ctrl Pts',(34.1763977434987,-72.5771484665379,-26.9980302481222));
#28016=CARTESIAN_POINT('Ctrl Pts',(34.1623275344883,-72.5706062766722,-26.9983500673599));
#28017=CARTESIAN_POINT('Ctrl Pts',(34.1490472500448,-72.5644337382725,-26.998615458806));
#28018=CARTESIAN_POINT('Ctrl Pts',(34.1371264940464,-72.5588930945864,-26.9988536816156));
#28019=CARTESIAN_POINT('Ctrl Pts',(34.1258429051091,-72.5536506163926,-26.999048201826));
#28020=CARTESIAN_POINT('Ctrl Pts',(34.1153205042047,-72.5487644340835,-26.9992071337772));
#28021=CARTESIAN_POINT('Ctrl Pts',(34.1054956763343,-72.5442021768033,-26.9993555294788));
#28022=CARTESIAN_POINT('Ctrl Pts',(34.0963348925316,-72.5399507407317,-26.9994729902421));
#28023=CARTESIAN_POINT('Ctrl Pts',(34.0879000947392,-72.5360390514954,-26.9995669997594));
#28024=CARTESIAN_POINT('Ctrl Pts',(34.0798812223448,-72.5323202502147,-26.9996563736059));
#28025=CARTESIAN_POINT('Ctrl Pts',(34.0725188196205,-72.5289086594304,-26.9997246070626));
#28026=CARTESIAN_POINT('Ctrl Pts',(34.0658243155296,-72.5258095023092,-26.9997779400933));
#28027=CARTESIAN_POINT('Ctrl Pts',(34.0593930548309,-72.5228322112176,-26.9998291759458));
#28028=CARTESIAN_POINT('Ctrl Pts',(34.0535784467592,-72.5201433779336,-26.9998666884134));
#28029=CARTESIAN_POINT('Ctrl Pts',(34.0483470066375,-72.5177272092184,-26.9998952450266));
#28030=CARTESIAN_POINT('Ctrl Pts',(34.0433636057174,-72.5154255987405,-26.99992244768));
#28031=CARTESIAN_POINT('Ctrl Pts',(34.038909464426,-72.5133714448828,-26.9999415292289));
#28032=CARTESIAN_POINT('Ctrl Pts',(34.0349130827146,-72.5115312156494,-26.999955676367));
#28033=CARTESIAN_POINT('Ctrl Pts',(34.0310069639009,-72.5097325501193,-26.9999695039757));
#28034=CARTESIAN_POINT('Ctrl Pts',(34.027538362589,-72.5081383474965,-26.9999786149847));
#28035=CARTESIAN_POINT('Ctrl Pts',(34.0243965595917,-72.506696796225,-26.999985050899));
#28036=CARTESIAN_POINT('Ctrl Pts',(34.0213534678907,-72.5053005365886,-26.9999912846053));
#28037=CARTESIAN_POINT('Ctrl Pts',(34.0186170471667,-72.5040475253501,-26.9999950010979));
#28038=CARTESIAN_POINT('Ctrl Pts',(34.0160430187993,-72.5028703359362,-26.9999972537214));
#28039=CARTESIAN_POINT('Ctrl Pts',(34.0138720346514,-72.5018774721476,-26.9999991536266));
#28040=CARTESIAN_POINT('Ctrl Pts',(34.0118159287574,-72.5009382459881,-27.));
#28041=CARTESIAN_POINT('Ctrl Pts',(34.0097619285762,-72.5,-27.));
#28042=CARTESIAN_POINT('',(38.6706975330488,-74.,-25.4999999993376));
#28043=CARTESIAN_POINT('Ctrl Pts',(38.670697532745,-74.,-25.4999999988754));
#28044=CARTESIAN_POINT('Ctrl Pts',(38.3641779127485,-74.0000000001514,-25.7018870729982));
#28045=CARTESIAN_POINT('Ctrl Pts',(37.5431082034452,-73.8929551961393,-26.1757552250324));
#28046=CARTESIAN_POINT('Ctrl Pts',(36.7538439760921,-73.6459407607355,-26.4950027398036));
#28047=CARTESIAN_POINT('Ctrl Pts',(35.7977539931684,-73.2955896700455,-26.7874092748223));
#28048=CARTESIAN_POINT('Ctrl Pts',(35.3787212463313,-73.1202082882644,-26.8774051537635));
#28049=CARTESIAN_POINT('Ctrl Pts',(34.9928690003034,-72.9498135639887,-26.9309674201923));
#28050=CARTESIAN_POINT('',(5.2,-74.,-25.5));
#28051=CARTESIAN_POINT('Origin',(-4.79999999999999,-32.,-20.));
#28052=CARTESIAN_POINT('',(-11.8,-32.,-20.));
#28053=CARTESIAN_POINT('Ctrl Pts',(-11.7309675556501,-72.9498131330638,
19.7928680244678));
#28054=CARTESIAN_POINT('Ctrl Pts',(-11.731923849979,-72.9467709227377,19.7859790576247));
#28055=CARTESIAN_POINT('Ctrl Pts',(-11.7337973388594,-72.9403543075767,
19.7715236532945));
#28056=CARTESIAN_POINT('Ctrl Pts',(-11.745649829374,-72.9035149361054,19.6878044517073));
#28057=CARTESIAN_POINT('Ctrl Pts',(-11.7734458065936,-72.7907458667152,
19.4364960250678));
#28058=CARTESIAN_POINT('Ctrl Pts',(-11.7924941021948,-72.6655779568151,
19.1664451757454));
#28059=CARTESIAN_POINT('Ctrl Pts',(-11.8001369161947,-72.5485936434818,
18.9151456492252));
#28060=CARTESIAN_POINT('Ctrl Pts',(-11.7998430894499,-72.5097905790976,
18.8311911012471));
#28061=CARTESIAN_POINT('Ctrl Pts',(-11.8,-72.5031610690666,18.8166823681909));
#28062=CARTESIAN_POINT('Ctrl Pts',(-11.8,-72.5,18.8097619285762));
#28063=CARTESIAN_POINT('Ctrl Pts',(-11.7529186757946,-72.648770667648,19.9322264436722));
#28064=CARTESIAN_POINT('Ctrl Pts',(-11.7533741068931,-72.646492978889,19.9271259487491));
#28065=CARTESIAN_POINT('Ctrl Pts',(-11.7541650463145,-72.6424667118156,
19.9181034609183));
#28066=CARTESIAN_POINT('Ctrl Pts',(-11.7623844804504,-72.6172317023529,
19.8602296711434));
#28067=CARTESIAN_POINT('Ctrl Pts',(-11.7851097685095,-72.5287894228312,
19.6622836986296));
#28068=CARTESIAN_POINT('Ctrl Pts',(-11.7974871269408,-72.4421791346063,
19.4764698099938));
#28069=CARTESIAN_POINT('Ctrl Pts',(-11.8015614206973,-72.3497074879145,
19.2786156236357));
#28070=CARTESIAN_POINT('Ctrl Pts',(-11.79999556323,-72.3228009293553,19.2206367739928));
#28071=CARTESIAN_POINT('Ctrl Pts',(-11.8,-72.3186768516068,19.2116122804521));
#28072=CARTESIAN_POINT('Ctrl Pts',(-11.8,-72.3163422783269,19.2065079523841));
#28073=CARTESIAN_POINT('Ctrl Pts',(-11.7748697959391,-72.3477282022321,
20.0715848628766));
#28074=CARTESIAN_POINT('Ctrl Pts',(-11.7750197265738,-72.3462456838324,
20.0683082748074));
#28075=CARTESIAN_POINT('Ctrl Pts',(-11.7755924033863,-72.3423623378614,
20.0597599762898));
#28076=CARTESIAN_POINT('Ctrl Pts',(-11.7789296771626,-72.3223173268409,
20.0158887345708));
#28077=CARTESIAN_POINT('Ctrl Pts',(-11.7857195676337,-72.2729882610716,
19.9084439154536));
#28078=CARTESIAN_POINT('Ctrl Pts',(-11.7947091257581,-72.207684036952,19.7662748679286));
#28079=CARTESIAN_POINT('Ctrl Pts',(-11.7983929922402,-72.1582937366765,
19.6589744106553));
#28080=CARTESIAN_POINT('Ctrl Pts',(-11.7997584237843,-72.1381225473783,
19.6151072341032));
#28081=CARTESIAN_POINT('Ctrl Pts',(-11.8,-72.134192634147,19.6065421927134));
#28082=CARTESIAN_POINT('Ctrl Pts',(-11.8,-72.1326845566538,19.6032539761921));
#28083=CARTESIAN_POINT('Ctrl Pts',(-11.7968209160836,-72.0466857368163,
20.210943282081));
#28084=CARTESIAN_POINT('Ctrl Pts',(-11.7968652729023,-72.0460043569062,
20.2094720016796));
#28085=CARTESIAN_POINT('Ctrl Pts',(-11.7969519847552,-72.044574118995,20.2063835827652));
#28086=CARTESIAN_POINT('Ctrl Pts',(-11.7975053588681,-72.0362657186926,
20.1884442076621));
#28087=CARTESIAN_POINT('Ctrl Pts',(-11.7987930795194,-72.0112738645727,
20.1344718117455));
#28088=CARTESIAN_POINT('Ctrl Pts',(-11.7996559734539,-71.9844301297503,
20.0764810684143));
#28089=CARTESIAN_POINT('Ctrl Pts',(-11.8000061189177,-71.9594531450371,
20.0225217914491));
#28090=CARTESIAN_POINT('Ctrl Pts',(-11.7999927847675,-71.9511381222097,
20.004560057106));
#28091=CARTESIAN_POINT('Ctrl Pts',(-11.8,-71.9497084166872,20.0014721049746));
#28092=CARTESIAN_POINT('Ctrl Pts',(-11.8,-71.9490268349807,20.));
#28093=CARTESIAN_POINT('',(-11.8,-72.5,18.8097619285762));
#28094=CARTESIAN_POINT('',(-11.7309675556501,-72.9498131330638,19.7928680244678));
#28095=CARTESIAN_POINT('Ctrl Pts',(-11.8,-72.5,18.8097619285762));
#28096=CARTESIAN_POINT('Ctrl Pts',(-11.8,-72.501104434069,18.8121798350255));
#28097=CARTESIAN_POINT('Ctrl Pts',(-11.799998844824,-72.5022107400032,18.8146017627203));
#28098=CARTESIAN_POINT('Ctrl Pts',(-11.7999961395225,-72.5034031482093,
18.8172080904455));
#28099=CARTESIAN_POINT('Ctrl Pts',(-11.7999933680139,-72.5046247382961,
18.8198782029923));
#28100=CARTESIAN_POINT('Ctrl Pts',(-11.7999889720745,-72.5059366396841,
18.8227417275941));
#28101=CARTESIAN_POINT('Ctrl Pts',(-11.7999817153247,-72.5074063278034,
18.8259430216939));
#28102=CARTESIAN_POINT('Ctrl Pts',(-11.7999742566232,-72.5089169166044,
18.8292334061994));
#28103=CARTESIAN_POINT('Ctrl Pts',(-11.7999637834255,-72.5105941315299,
18.83288047915));
#28104=CARTESIAN_POINT('Ctrl Pts',(-11.7999480152244,-72.5124880592726,
18.8369912426304));
#28105=CARTESIAN_POINT('Ctrl Pts',(-11.799931738317,-72.5144430880226,18.8412346256316));
#28106=CARTESIAN_POINT('Ctrl Pts',(-11.7999098218899,-72.5166289622411,
18.8459719331802));
#28107=CARTESIAN_POINT('Ctrl Pts',(-11.7998786784034,-72.5190774754851,
18.8512709182692));
#28108=CARTESIAN_POINT('Ctrl Pts',(-11.7998456108804,-72.5216772572391,
18.856897273276));
#28109=CARTESIAN_POINT('Ctrl Pts',(-11.7998021319534,-72.5245731226337,
18.8631568226208));
#28110=CARTESIAN_POINT('Ctrl Pts',(-11.7997427762118,-72.5277777824963,
18.8700764316877));
#28111=CARTESIAN_POINT('Ctrl Pts',(-11.7996802900758,-72.5311514546459,
18.8773609777534));
#28112=CARTESIAN_POINT('Ctrl Pts',(-11.7996001669453,-72.5348672363336,
18.8853767852421));
#28113=CARTESIAN_POINT('Ctrl Pts',(-11.7994951564366,-72.5389136971142,
18.8940991505868));
#28114=CARTESIAN_POINT('Ctrl Pts',(-11.7993826824823,-72.5432477533008,
18.9034414434036));
#28115=CARTESIAN_POINT('Ctrl Pts',(-11.7992415706987,-72.5479610044147,
18.9135939447027));
#28116=CARTESIAN_POINT('Ctrl Pts',(-11.7990629471554,-72.5530120784887,
18.9244681723169));
#28117=CARTESIAN_POINT('Ctrl Pts',(-11.7988649429092,-72.558611195469,18.936522256575));
#28118=CARTESIAN_POINT('Ctrl Pts',(-11.7986206702861,-72.5646251589742,
18.9494626076275));
#28119=CARTESIAN_POINT('Ctrl Pts',(-11.7983202304374,-72.57096821163,18.9631064122645));
#28120=CARTESIAN_POINT('Ctrl Pts',(-11.7979524431966,-72.5787331397677,
18.9798086482823));
#28121=CARTESIAN_POINT('Ctrl Pts',(-11.7974999722516,-72.5869905301776,
18.9975635488976));
#28122=CARTESIAN_POINT('Ctrl Pts',(-11.7969538016201,-72.5955474532106,
19.0159607182475));
#28123=CARTESIAN_POINT('Ctrl Pts',(-11.7963926885023,-72.6043384820302,
19.0348612091517));
#28124=CARTESIAN_POINT('Ctrl Pts',(-11.7957325786725,-72.6134430509656,
19.0544340658146));
#28125=CARTESIAN_POINT('Ctrl Pts',(-11.7949775407195,-72.6226464542671,
19.0742232187693));
#28126=CARTESIAN_POINT('Ctrl Pts',(-11.7943746852057,-72.629994856297,19.0900237489622));
#28127=CARTESIAN_POINT('Ctrl Pts',(-11.7937117025217,-72.6374056335299,
19.1059608261794));
#28128=CARTESIAN_POINT('Ctrl Pts',(-11.7929961401608,-72.6447844102966,
19.1218342983521));
#28129=CARTESIAN_POINT('Ctrl Pts',(-11.792357485478,-72.6513701260821,19.136001711131));
#28130=CARTESIAN_POINT('Ctrl Pts',(-11.7916771251311,-72.6579301278489,
19.1501179668206));
#28131=CARTESIAN_POINT('Ctrl Pts',(-11.7909619574117,-72.6644154541125,
19.1640797110818));
#28132=CARTESIAN_POINT('Ctrl Pts',(-11.7902956522372,-72.6704576821541,
19.1770875443434));
#28133=CARTESIAN_POINT('Ctrl Pts',(-11.7895992563685,-72.6764349461207,
19.1899609298704));
#28134=CARTESIAN_POINT('Ctrl Pts',(-11.7888777417671,-72.6823268221364,
19.2026576733767));
#28135=CARTESIAN_POINT('Ctrl Pts',(-11.7881926293819,-72.6879214382716,
19.2147138344186));
#28136=CARTESIAN_POINT('Ctrl Pts',(-11.7874849648868,-72.6934389605026,
19.226610481107));
#28137=CARTESIAN_POINT('Ctrl Pts',(-11.7867569121391,-72.6988815833769,
19.2383542485831));
#28138=CARTESIAN_POINT('Ctrl Pts',(-11.7860580430633,-72.7041060411245,
19.2496272723425));
#28139=CARTESIAN_POINT('Ctrl Pts',(-11.7853404669398,-72.7092614026539,
19.2607592299266));
#28140=CARTESIAN_POINT('Ctrl Pts',(-11.7846028726666,-72.7143695651672,
19.2717996399125));
#28141=CARTESIAN_POINT('Ctrl Pts',(-11.783851133165,-72.7195756895665,19.2830517775755));
#28142=CARTESIAN_POINT('Ctrl Pts',(-11.7830787256541,-72.7247325197476,
19.2942082079411));
#28143=CARTESIAN_POINT('Ctrl Pts',(-11.782279253214,-72.7298873974176,19.305374569448));
#28144=CARTESIAN_POINT('Ctrl Pts',(-11.7815108442834,-72.7348419822645,
19.3161070618677));
#28145=CARTESIAN_POINT('Ctrl Pts',(-11.7807168472023,-72.7397983610911,
19.3268566425138));
#28146=CARTESIAN_POINT('Ctrl Pts',(-11.7798905612536,-72.7447936410788,
19.3377066031678));
#28147=CARTESIAN_POINT('Ctrl Pts',(-11.7790348821557,-72.7499666162216,
19.3489425252584));
#28148=CARTESIAN_POINT('Ctrl Pts',(-11.7781445235792,-72.7551812136779,
19.3602859041663));
#28149=CARTESIAN_POINT('Ctrl Pts',(-11.7772145611532,-72.7604556398259,
19.3717788059764));
#28150=CARTESIAN_POINT('Ctrl Pts',(-11.7762202119557,-72.7660952455349,
19.3840674290118));
#28151=CARTESIAN_POINT('Ctrl Pts',(-11.7751805066769,-72.7718032174321,
19.3965269512495));
#28152=CARTESIAN_POINT('Ctrl Pts',(-11.7740933204493,-72.7775768048788,
19.409153596826));
#28153=CARTESIAN_POINT('Ctrl Pts',(-11.7729402752532,-72.7837001415264,
19.4225451323848));
#28154=CARTESIAN_POINT('Ctrl Pts',(-11.7717337402544,-72.7898971149349,
19.4361243256637));
#28155=CARTESIAN_POINT('Ctrl Pts',(-11.7704767177068,-72.7961388570963,
19.4498295830909));
#28156=CARTESIAN_POINT('Ctrl Pts',(-11.7691117732257,-72.8029164853351,
19.4647115082578));
#28157=CARTESIAN_POINT('Ctrl Pts',(-11.7676871916452,-72.8097466432146,
19.479741585126));
#28158=CARTESIAN_POINT('Ctrl Pts',(-11.766214782111,-72.8165662848746,19.4947816596443));
#28159=CARTESIAN_POINT('Ctrl Pts',(-11.7645116079786,-72.8244547404956,
19.51217890224));
#28160=CARTESIAN_POINT('Ctrl Pts',(-11.7627442453546,-72.8323286372044,
19.5295886154485));
#28161=CARTESIAN_POINT('Ctrl Pts',(-11.7609440847192,-72.8400623197651,
19.5467306475706));
#28162=CARTESIAN_POINT('Ctrl Pts',(-11.7585963565591,-72.8501484109567,
19.5690868921974));
#28163=CARTESIAN_POINT('Ctrl Pts',(-11.7561926064093,-72.8599933687506,
19.5909825486672));
#28164=CARTESIAN_POINT('Ctrl Pts',(-11.7538294614589,-72.8692964892794,
19.6117338510281));
#28165=CARTESIAN_POINT('Ctrl Pts',(-11.7521606565975,-72.8758661636289,
19.6263879983561));
#28166=CARTESIAN_POINT('Ctrl Pts',(-11.750512913278,-72.8821649104921,19.6404694774992));
#28167=CARTESIAN_POINT('Ctrl Pts',(-11.7489236489795,-72.8880982600167,
19.6537587709998));
#28168=CARTESIAN_POINT('Ctrl Pts',(-11.7474976601362,-72.8934220379643,
19.6656827689681));
#28169=CARTESIAN_POINT('Ctrl Pts',(-11.746118990168,-72.8984513774563,19.6769682936816));
#28170=CARTESIAN_POINT('Ctrl Pts',(-11.7448124401235,-72.9031339887237,
19.6874909539757));
#28171=CARTESIAN_POINT('Ctrl Pts',(-11.7435926877885,-72.9075055212583,
19.6973145650337));
#28172=CARTESIAN_POINT('Ctrl Pts',(-11.7424359361705,-72.9115747003093,
19.7064728666794));
#28173=CARTESIAN_POINT('Ctrl Pts',(-11.7413577511394,-72.9153165458182,
19.7149037671804));
#28174=CARTESIAN_POINT('Ctrl Pts',(-11.7403328121501,-72.9188736007237,
19.722918308645));
#28175=CARTESIAN_POINT('Ctrl Pts',(-11.7393789657513,-72.9221347341473,
19.7302752031999));
#28176=CARTESIAN_POINT('Ctrl Pts',(-11.7385035999542,-72.925096921794,19.7369630176401));
#28177=CARTESIAN_POINT('Ctrl Pts',(-11.7376626969175,-72.9279424894366,
19.743387535814));
#28178=CARTESIAN_POINT('Ctrl Pts',(-11.7368942766262,-72.9305120885608,
19.7491943710544));
#28179=CARTESIAN_POINT('Ctrl Pts',(-11.7361981280593,-72.9328220615438,
19.7544171202232));
#28180=CARTESIAN_POINT('Ctrl Pts',(-11.7355350110767,-72.935022428516,19.7593920549342));
#28181=CARTESIAN_POINT('Ctrl Pts',(-11.7349374860318,-72.9369871912694,
19.7638369366522));
#28182=CARTESIAN_POINT('Ctrl Pts',(-11.7343986079509,-72.9387489413189,
19.7678234681457));
#28183=CARTESIAN_POINT('Ctrl Pts',(-11.73387191165,-72.940470865567,19.7717198808326));
#28184=CARTESIAN_POINT('Ctrl Pts',(-11.7334012661809,-72.9419987635744,
19.7751782288516));
#28185=CARTESIAN_POINT('Ctrl Pts',(-11.7329732356419,-72.9433821218023,
19.7783095280656));
#28186=CARTESIAN_POINT('Ctrl Pts',(-11.7325586563635,-72.9447220067026,
19.7813424232698));
#28187=CARTESIAN_POINT('Ctrl Pts',(-11.7321840603972,-72.9459262548977,
19.7840684168231));
#28188=CARTESIAN_POINT('Ctrl Pts',(-11.7318304518762,-72.9470587848148,
19.7866321657248));
#28189=CARTESIAN_POINT('Ctrl Pts',(-11.7315331756714,-72.9480108947768,
19.788787491454));
#28190=CARTESIAN_POINT('Ctrl Pts',(-11.7312506313311,-72.948912598852,19.7908287998052));
#28191=CARTESIAN_POINT('Ctrl Pts',(-11.7309675556501,-72.9498131330638,
19.7928680244678));
#28192=CARTESIAN_POINT('',(-11.7968209160836,-72.0466857368163,20.210943282081));
#28193=CARTESIAN_POINT('Ctrl Pts',(-11.7968209160836,-72.0466857368163,
20.210943282081));
#28194=CARTESIAN_POINT('Ctrl Pts',(-11.7748697959391,-72.3477282022321,
20.0715848628766));
#28195=CARTESIAN_POINT('Ctrl Pts',(-11.7529186757946,-72.648770667648,19.9322264436722));
#28196=CARTESIAN_POINT('Ctrl Pts',(-11.7309675556501,-72.9498131330638,
19.7928680244678));
#28197=CARTESIAN_POINT('',(-11.8,-71.9490268349807,20.));
#28198=CARTESIAN_POINT('Ctrl Pts',(-11.7968209160836,-72.0466857368163,
20.210943282081));
#28199=CARTESIAN_POINT('Ctrl Pts',(-11.7968440264343,-72.0463307309993,
20.2101767301277));
#28200=CARTESIAN_POINT('Ctrl Pts',(-11.796867151744,-72.0459737810207,20.2094059772171));
#28201=CARTESIAN_POINT('Ctrl Pts',(-11.7968938349779,-72.0455591055399,
20.2085105801841));
#28202=CARTESIAN_POINT('Ctrl Pts',(-11.7969215748069,-72.0451280098565,
20.2075797274724));
#28203=CARTESIAN_POINT('Ctrl Pts',(-11.7969531556842,-72.0446346198902,
20.2065143654833));
#28204=CARTESIAN_POINT('Ctrl Pts',(-11.7969907706432,-72.0440407131694,
20.2052319554395));
#28205=CARTESIAN_POINT('Ctrl Pts',(-11.7970302352795,-72.0434176016909,
20.2038864841889));
#28206=CARTESIAN_POINT('Ctrl Pts',(-11.7970763351041,-72.0426839627647,
20.2023023485085));
#28207=CARTESIAN_POINT('Ctrl Pts',(-11.7971297471362,-72.0418204588819,
20.2004377752349));
#28208=CARTESIAN_POINT('Ctrl Pts',(-11.7971866204212,-72.0409009974715,
20.1984523722666));
#28209=CARTESIAN_POINT('Ctrl Pts',(-11.7972517663276,-72.039834454825,20.1961493535317));
#28210=CARTESIAN_POINT('Ctrl Pts',(-11.7973241283667,-72.0386228526127,
20.1935330529333));
#28211=CARTESIAN_POINT('Ctrl Pts',(-11.7974033531205,-72.0372963437394,
20.1906686260414));
#28212=CARTESIAN_POINT('Ctrl Pts',(-11.7974911870066,-72.0357962057728,
20.1874292153278));
#28213=CARTESIAN_POINT('Ctrl Pts',(-11.797584514987,-72.0341515121678,20.1838775560358));
#28214=CARTESIAN_POINT('Ctrl Pts',(-11.7976993757062,-72.0321273529657,
20.1795064538339));
#28215=CARTESIAN_POINT('Ctrl Pts',(-11.7978224459019,-72.0298846925149,
20.1746633732519));
#28216=CARTESIAN_POINT('Ctrl Pts',(-11.7979466024095,-72.0275116964433,
20.1695386381506));
#28217=CARTESIAN_POINT('Ctrl Pts',(-11.7980821533145,-72.0249209199172,
20.1639435832067));
#28218=CARTESIAN_POINT('Ctrl Pts',(-11.7982187728114,-72.0221774130801,
20.158018473028));
#28219=CARTESIAN_POINT('Ctrl Pts',(-11.7983487795842,-72.0194065699847,
20.1520340728002));
#28220=CARTESIAN_POINT('Ctrl Pts',(-11.7984473485597,-72.0173057627787,
20.1474967999597));
#28221=CARTESIAN_POINT('Ctrl Pts',(-11.798542156045,-72.0151898308566,20.1429267194323));
#28222=CARTESIAN_POINT('Ctrl Pts',(-11.798631372502,-72.0131013188954,20.1384157210412));
#28223=CARTESIAN_POINT('Ctrl Pts',(-11.7987118838834,-72.0112165883329,
20.1343448721818));
#28224=CARTESIAN_POINT('Ctrl Pts',(-11.7987878612489,-72.0093544513597,
20.1303227080409));
#28225=CARTESIAN_POINT('Ctrl Pts',(-11.798859022311,-72.0075300311517,20.1263819046227));
#28226=CARTESIAN_POINT('Ctrl Pts',(-11.7989256149733,-72.0058227351215,
20.1226940930084));
#28227=CARTESIAN_POINT('Ctrl Pts',(-11.7989880057221,-72.0041486403605,
20.1190779023675));
#28228=CARTESIAN_POINT('Ctrl Pts',(-11.7990467044472,-72.0025022857801,
20.1155215519588));
#28229=CARTESIAN_POINT('Ctrl Pts',(-11.7991060919784,-72.0008366118854,
20.1119234691965));
#28230=CARTESIAN_POINT('Ctrl Pts',(-11.799161711364,-71.9991997282623,20.1083874932517));
#28231=CARTESIAN_POINT('Ctrl Pts',(-11.7992146913247,-71.997562572897,20.1048508690689));
#28232=CARTESIAN_POINT('Ctrl Pts',(-11.7992663579433,-71.9959660016519,
20.1014019157228));
#28233=CARTESIAN_POINT('Ctrl Pts',(-11.79931563984,-71.9943651666199,20.0979436948263));
#28234=CARTESIAN_POINT('Ctrl Pts',(-11.7993631272831,-71.9927356970362,
20.0944235798376));
#28235=CARTESIAN_POINT('Ctrl Pts',(-11.7994134018494,-71.991010590962,20.090696862991));
#28236=CARTESIAN_POINT('Ctrl Pts',(-11.7994616361791,-71.9892535447088,
20.0869011062902));
#28237=CARTESIAN_POINT('Ctrl Pts',(-11.7995075723881,-71.987460970195,20.0830285738881));
#28238=CARTESIAN_POINT('Ctrl Pts',(-11.7995572904833,-71.9855208146535,
20.0788372194189));
#28239=CARTESIAN_POINT('Ctrl Pts',(-11.7996042772797,-71.9835392694514,
20.0745564223789));
#28240=CARTESIAN_POINT('Ctrl Pts',(-11.7996476627856,-71.9815377443596,
20.0702324487684));
#28241=CARTESIAN_POINT('Ctrl Pts',(-11.7996984016496,-71.9791969831453,
20.0651756099806));
#28242=CARTESIAN_POINT('Ctrl Pts',(-11.7997441440131,-71.9768292652326,
20.0600605172037));
#28243=CARTESIAN_POINT('Ctrl Pts',(-11.7997837204606,-71.9744988699031,
20.0550260554206));
#28244=CARTESIAN_POINT('Ctrl Pts',(-11.799841617981,-71.9710896677201,20.0476609968471));
#28245=CARTESIAN_POINT('Ctrl Pts',(-11.7998859839155,-71.967763829697,20.0404760377697));
#28246=CARTESIAN_POINT('Ctrl Pts',(-11.799917487043,-71.9647604963972,20.0339878594497));
#28247=CARTESIAN_POINT('Ctrl Pts',(-11.7999376069614,-71.9628423750572,
20.0298440924912));
#28248=CARTESIAN_POINT('Ctrl Pts',(-11.7999526242593,-71.9610565580338,
20.0259861725226));
#28249=CARTESIAN_POINT('Ctrl Pts',(-11.7999637788496,-71.9594514906785,
20.0225187653674));
#28250=CARTESIAN_POINT('Ctrl Pts',(-11.7999740893287,-71.9579678850111,
20.0193137503941));
#28251=CARTESIAN_POINT('Ctrl Pts',(-11.7999811326703,-71.9566391654818,
20.0164433694765));
#28252=CARTESIAN_POINT('Ctrl Pts',(-11.7999861098761,-71.9554826093196,
20.013944946831));
#28253=CARTESIAN_POINT('Ctrl Pts',(-11.7999904546681,-71.9544730074948,
20.0117639787601));
#28254=CARTESIAN_POINT('Ctrl Pts',(-11.7999932364772,-71.9535945583468,
20.0098663653902));
#28255=CARTESIAN_POINT('Ctrl Pts',(-11.7999951540824,-71.9528401206129,
20.0082366754872));
#28256=CARTESIAN_POINT('Ctrl Pts',(-11.7999969972036,-71.952114986876,20.006670286273));
#28257=CARTESIAN_POINT('Ctrl Pts',(-11.7999980448829,-71.9515045768435,
20.0053517545772));
#28258=CARTESIAN_POINT('Ctrl Pts',(-11.7999987249728,-71.9509829203972,
20.0042249709247));
#28259=CARTESIAN_POINT('Ctrl Pts',(-11.7999993730205,-71.9504858415435,
20.0031512751423));
#28260=CARTESIAN_POINT('Ctrl Pts',(-11.7999996854038,-71.9500694193736,
20.0022518343659));
#28261=CARTESIAN_POINT('Ctrl Pts',(-11.7999998528112,-71.9496914618382,
20.0014354939551));
#28262=CARTESIAN_POINT('Ctrl Pts',(-11.7999999551045,-71.9494605131145,
20.0009366739598));
#28263=CARTESIAN_POINT('Ctrl Pts',(-11.8,-71.9492435363226,20.0004680394447));
#28264=CARTESIAN_POINT('Ctrl Pts',(-11.8,-71.9490268349807,20.));
#28265=CARTESIAN_POINT('',(-11.8,-72.2245134174903,19.4048809642881));
#28266=CARTESIAN_POINT('Ctrl Pts',(-5.01094426619173,-72.0466861925674,
26.9968208864141));
#28267=CARTESIAN_POINT('Ctrl Pts',(-5.00947297646683,-72.0460048083194,
26.996865243721));
#28268=CARTESIAN_POINT('Ctrl Pts',(-5.0063845384978,-72.0445745615206,26.9969519565246));
#28269=CARTESIAN_POINT('Ctrl Pts',(-4.98844507070461,-72.0362661183909,
26.9975053360185));
#28270=CARTESIAN_POINT('Ctrl Pts',(-4.93447244718678,-72.0112741569711,
26.9987930679778));
#28271=CARTESIAN_POINT('Ctrl Pts',(-4.87648146296461,-71.984430300943,26.9996559698239));
#28272=CARTESIAN_POINT('Ctrl Pts',(-4.82252191221301,-71.9594531916436,
27.0000061189759));
#28273=CARTESIAN_POINT('Ctrl Pts',(-4.80456008230516,-71.951138130719,26.9999927846913));
#28274=CARTESIAN_POINT('Ctrl Pts',(-4.80147211312516,-71.9497084193948,
27.));
#28275=CARTESIAN_POINT('Ctrl Pts',(-4.8,-71.9490268349807,27.));
#28276=CARTESIAN_POINT('Ctrl Pts',(-4.87158584422818,-72.3477286497075,
26.974869731007));
#28277=CARTESIAN_POINT('Ctrl Pts',(-4.86830922557782,-72.3462461176065,
26.9750196643687));
#28278=CARTESIAN_POINT('Ctrl Pts',(-4.85975897842875,-72.3423627521791,
26.9755114207066));
#28279=CARTESIAN_POINT('Ctrl Pts',(-4.81591321368326,-72.3223177067783,
26.9782702084194));
#28280=CARTESIAN_POINT('Ctrl Pts',(-4.70857333101532,-72.272988635298,26.9845161337709));
#28281=CARTESIAN_POINT('Ctrl Pts',(-4.56639009565372,-72.2076844178794,
26.9930985489782));
#28282=CARTESIAN_POINT('Ctrl Pts',(-4.45903094371778,-72.1582940094813,
26.9980897400517));
#28283=CARTESIAN_POINT('Ctrl Pts',(-4.41511199664308,-72.138122656842,26.9997839104599));
#28284=CARTESIAN_POINT('Ctrl Pts',(-4.40654219803927,-72.1341926745702,
27.));
#28285=CARTESIAN_POINT('Ctrl Pts',(-4.40325397619206,-72.1326845566538,
27.));
#28286=CARTESIAN_POINT('Ctrl Pts',(-4.73222742226463,-72.6487711068476,
26.9529185755998));
#28287=CARTESIAN_POINT('Ctrl Pts',(-4.72712687588195,-72.646493395594,26.9533740167535));
#28288=CARTESIAN_POINT('Ctrl Pts',(-4.71810428296693,-72.6425801839039,
26.9544902505489));
#28289=CARTESIAN_POINT('Ctrl Pts',(-4.66023026081951,-72.6159497943818,
26.962298209812));
#28290=CARTESIAN_POINT('Ctrl Pts',(-4.46228446583122,-72.5231679093969,
26.9782325012995));
#28291=CARTESIAN_POINT('Ctrl Pts',(-4.2764703099712,-72.4384023248246,26.9937562016165));
#28292=CARTESIAN_POINT('Ctrl Pts',(-4.07861571985972,-72.3480976161143,
26.9979643889596));
#28293=CARTESIAN_POINT('Ctrl Pts',(-4.02063678651915,-72.3226743264951,
26.9994070919264));
#28294=CARTESIAN_POINT('Ctrl Pts',(-4.01161228295339,-72.3186769297456,
27.));
#28295=CARTESIAN_POINT('Ctrl Pts',(-4.00650795238413,-72.3163422783269,
27.));
#28296=CARTESIAN_POINT('Ctrl Pts',(-4.59286900030108,-72.9498135639877,
26.9309674201926));
#28297=CARTESIAN_POINT('Ctrl Pts',(-4.5859799608391,-72.9467713218037,26.9319237255424));
#28298=CARTESIAN_POINT('Ctrl Pts',(-4.57152441475369,-72.9403546462486,
26.933797234493));
#28299=CARTESIAN_POINT('Ctrl Pts',(-4.48780490143884,-72.9035150752116,
26.9456497972286));
#28300=CARTESIAN_POINT('Ctrl Pts',(-4.23649663915558,-72.7907461114549,
26.9734457309761));
#28301=CARTESIAN_POINT('Ctrl Pts',(-3.96644557228501,-72.665579292086,26.9924939338067));
#28302=CARTESIAN_POINT('Ctrl Pts',(-3.71514570094186,-72.5485946771508,
27.0001369006243));
#28303=CARTESIAN_POINT('Ctrl Pts',(-3.63119110304352,-72.5097909222079,
26.9998430866664));
#28304=CARTESIAN_POINT('Ctrl Pts',(-3.6166823678675,-72.503161184921,27.));
#28305=CARTESIAN_POINT('Ctrl Pts',(-3.60976192857619,-72.5,27.));
#28306=CARTESIAN_POINT('',(-4.8,-71.9490268349807,27.));
#28307=CARTESIAN_POINT('',(-5.01094426619173,-72.0466861925674,26.9968208864141));
#28308=CARTESIAN_POINT('Ctrl Pts',(-4.8,-71.9490268349807,27.));
#28309=CARTESIAN_POINT('Ctrl Pts',(-4.80076697070348,-71.9493819403517,
27.));
#28310=CARTESIAN_POINT('Ctrl Pts',(-4.80153814101389,-71.9497389896615,
26.9999998883361));
#28311=CARTESIAN_POINT('Ctrl Pts',(-4.80243401101288,-71.9501537584991,
26.9999995768279));
#28312=CARTESIAN_POINT('Ctrl Pts',(-4.8033653543852,-71.9505849507574,26.999999252985));
#28313=CARTESIAN_POINT('Ctrl Pts',(-4.80443126675711,-71.9510784307137,
26.999998715007));
#28314=CARTESIAN_POINT('Ctrl Pts',(-4.80571431921969,-71.9516724170336,
26.9999976676107));
#28315=CARTESIAN_POINT('Ctrl Pts',(-4.80706046220201,-71.9522956109712,
26.9999965687117));
#28316=CARTESIAN_POINT('Ctrl Pts',(-4.80864537002902,-71.9530293205579,
26.9999949098187));
#28317=CARTESIAN_POINT('Ctrl Pts',(-4.81051081979623,-71.953892881673,26.9999921087575));
#28318=CARTESIAN_POINT('Ctrl Pts',(-4.81249715032639,-71.9548124013714,
26.9999891261881));
#28319=CARTESIAN_POINT('Ctrl Pts',(-4.81480121272597,-71.9558789862512,
26.9999848410617));
#28320=CARTESIAN_POINT('Ctrl Pts',(-4.81741864449946,-71.9570906156706,
26.9999783278824));
#28321=CARTESIAN_POINT('Ctrl Pts',(-4.82028429268157,-71.958417146386,26.9999711970451));
#28322=CARTESIAN_POINT('Ctrl Pts',(-4.82352502414162,-71.9599172861368,
26.9999613711321));
#28323=CARTESIAN_POINT('Ctrl Pts',(-4.82707803879157,-71.9615619664985,
26.9999476269337));
#28324=CARTESIAN_POINT('Ctrl Pts',(-4.83145062144543,-71.9635860225549,
26.9999307123839));
#28325=CARTESIAN_POINT('Ctrl Pts',(-4.83629519151344,-71.9658285383687,
26.9999077806186));
#28326=CARTESIAN_POINT('Ctrl Pts',(-4.84142131794206,-71.9682013731942,
26.9998774471001));
#28327=CARTESIAN_POINT('Ctrl Pts',(-4.84701870318713,-71.9707923492121,
26.9998443249382));
#28328=CARTESIAN_POINT('Ctrl Pts',(-4.85294611909829,-71.9735360807744,
26.9998023221268));
#28329=CARTESIAN_POINT('Ctrl Pts',(-4.85893259038397,-71.9763071508735,
26.9997519205891));
#28330=CARTESIAN_POINT('Ctrl Pts',(-4.86347111047887,-71.9784079806827,
26.9997137096998));
#28331=CARTESIAN_POINT('Ctrl Pts',(-4.86804230004885,-71.9805239342998,
26.9996707497673));
#28332=CARTESIAN_POINT('Ctrl Pts',(-4.87255423493374,-71.9826124675569,
26.9996239815431));
#28333=CARTESIAN_POINT('Ctrl Pts',(-4.87662590506207,-71.9844972062981,
26.9995817768601));
#28334=CARTESIAN_POINT('Ctrl Pts',(-4.88064875130215,-71.9863593514082,
26.9995365071788));
#28335=CARTESIAN_POINT('Ctrl Pts',(-4.88459008953543,-71.9881837792468,
26.9994888753931));
#28336=CARTESIAN_POINT('Ctrl Pts',(-4.88827839296645,-71.9898910784073,
26.9994443015788));
#28337=CARTESIAN_POINT('Ctrl Pts',(-4.89189494739972,-71.9915651760262,
26.9993976862506));
#28338=CARTESIAN_POINT('Ctrl Pts',(-4.89545153213979,-71.9932115313249,
26.9993491843894));
#28339=CARTESIAN_POINT('Ctrl Pts',(-4.8990489039423,-71.9948767670949,26.9993001263068));
#28340=CARTESIAN_POINT('Ctrl Pts',(-4.902584072253,-71.9965132267009,26.9992491748664));
#28341=CARTESIAN_POINT('Ctrl Pts',(-4.90611972984301,-71.9981499419667,
26.9991955682734));
#28342=CARTESIAN_POINT('Ctrl Pts',(-4.90956865163276,-71.9997465057742,
26.9991432767429));
#28343=CARTESIAN_POINT('Ctrl Pts',(-4.91302668987658,-72.0013473181756,
26.9990883234737));
#28344=CARTESIAN_POINT('Ctrl Pts',(-4.91654648739712,-72.002976758872,26.999029712487));
#28345=CARTESIAN_POINT('Ctrl Pts',(-4.92027284370588,-72.0047018230506,
26.9989676619233));
#28346=CARTESIAN_POINT('Ctrl Pts',(-4.924068087188,-72.0064588199744,26.9989014928217));
#28347=CARTESIAN_POINT('Ctrl Pts',(-4.92793996922138,-72.0082513459319,
26.9988307140747));
#28348=CARTESIAN_POINT('Ctrl Pts',(-4.9321305670819,-72.0101914245235,26.9987541091412));
#28349=CARTESIAN_POINT('Ctrl Pts',(-4.93641044374858,-72.0121728926472,
26.9986720801898));
#28350=CARTESIAN_POINT('Ctrl Pts',(-4.94073336345865,-72.0141743492429,
26.9985851513295));
#28351=CARTESIAN_POINT('Ctrl Pts',(-4.94578880707783,-72.0165149550498,
26.99848349227));
#28352=CARTESIAN_POINT('Ctrl Pts',(-4.95090231692142,-72.0188825276485,
26.9983750851362));
#28353=CARTESIAN_POINT('Ctrl Pts',(-4.95593510268464,-72.021212804208,26.9982629447421));
#28354=CARTESIAN_POINT('Ctrl Pts',(-4.96329866291305,-72.0246222741522,
26.9980988700954));
#28355=CARTESIAN_POINT('Ctrl Pts',(-4.97048187721421,-72.0279484172632,
26.9979266950891));
#28356=CARTESIAN_POINT('Ctrl Pts',(-4.9769682776892,-72.030952030051,26.9977626587854));
#28357=CARTESIAN_POINT('Ctrl Pts',(-4.9811109071306,-72.0328703289307,26.9976578947297));
#28358=CARTESIAN_POINT('Ctrl Pts',(-4.98496767933264,-72.0346563122562,
26.9975566436896));
#28359=CARTESIAN_POINT('Ctrl Pts',(-4.98843399270563,-72.0362615170322,
26.9974632996818));
#28360=CARTESIAN_POINT('Ctrl Pts',(-4.99163799870267,-72.0377452506638,
26.9973770193232));
#28361=CARTESIAN_POINT('Ctrl Pts',(-4.99450741737523,-72.0390740730504,
26.9972975574334));
#28362=CARTESIAN_POINT('Ctrl Pts',(-4.99700496260522,-72.040230697167,26.9972272397507));
#28363=CARTESIAN_POINT('Ctrl Pts',(-4.99918507340499,-72.041240316011,26.997165859345));
#28364=CARTESIAN_POINT('Ctrl Pts',(-5.00108191836741,-72.0421187666742,
26.9971114553097));
#28365=CARTESIAN_POINT('Ctrl Pts',(-5.00271093426901,-72.0428731874743,
26.9970642613262));
#28366=CARTESIAN_POINT('Ctrl Pts',(-5.00427667108349,-72.0435983028148,
26.9970189005919));
#28367=CARTESIAN_POINT('Ctrl Pts',(-5.00559463926482,-72.0442086780512,
26.9969802139162));
#28368=CARTESIAN_POINT('Ctrl Pts',(-5.00672092624159,-72.0447302826953,
26.9969469383906));
#28369=CARTESIAN_POINT('Ctrl Pts',(-5.00779414404587,-72.0452273100093,
26.9969152307644));
#28370=CARTESIAN_POINT('Ctrl Pts',(-5.0086931690725,-72.0456436659006,26.9968884389805));
#28371=CARTESIAN_POINT('Ctrl Pts',(-5.00950910963114,-72.0460215435603,
26.9968640070378));
#28372=CARTESIAN_POINT('Ctrl Pts',(-5.01000782568555,-72.0462525084922,
26.9968490738397));
#28373=CARTESIAN_POINT('Ctrl Pts',(-5.01047634434494,-72.0464694884266,
26.9968349935968));
#28374=CARTESIAN_POINT('Ctrl Pts',(-5.01094426619173,-72.0466861925674,
26.9968208864141));
#28375=CARTESIAN_POINT('',(-4.59286900030108,-72.9498135639877,26.9309674201926));
#28376=CARTESIAN_POINT('Ctrl Pts',(-4.59286900030108,-72.9498135639877,
26.9309674201926));
#28377=CARTESIAN_POINT('Ctrl Pts',(-4.73222742226463,-72.6487711068476,
26.9529185755998));
#28378=CARTESIAN_POINT('Ctrl Pts',(-4.87158584422818,-72.3477286497075,
26.974869731007));
#28379=CARTESIAN_POINT('Ctrl Pts',(-5.01094426619173,-72.0466861925674,
26.9968208864141));
#28380=CARTESIAN_POINT('',(-3.60976192857619,-72.5,27.));
#28381=CARTESIAN_POINT('Ctrl Pts',(-4.59286900030109,-72.9498135639877,
26.9309674201926));
#28382=CARTESIAN_POINT('Ctrl Pts',(-4.5904606339385,-72.948750014594,26.9313017387358));
#28383=CARTESIAN_POINT('Ctrl Pts',(-4.58804823665763,-72.9476843461918,
26.9316354879945));
#28384=CARTESIAN_POINT('Ctrl Pts',(-4.58545108096436,-72.9465370382974,
26.9319932518796));
#28385=CARTESIAN_POINT('Ctrl Pts',(-4.58279030740325,-72.945361626858,26.9323597792652));
#28386=CARTESIAN_POINT('Ctrl Pts',(-4.57993573759051,-72.9441005819349,
26.9327514972647));
#28387=CARTESIAN_POINT('Ctrl Pts',(-4.57674274787858,-72.9426899331027,
26.9331872254278));
#28388=CARTESIAN_POINT('Ctrl Pts',(-4.57346080562075,-72.9412399854263,
26.9336350924116));
#28389=CARTESIAN_POINT('Ctrl Pts',(-4.56982146787799,-72.9396320460181,
26.9341294433979));
#28390=CARTESIAN_POINT('Ctrl Pts',(-4.56571755385512,-72.9378182307471,
26.9346829603872));
#28391=CARTESIAN_POINT('Ctrl Pts',(-4.56148107948029,-72.9359458275064,
26.9352543565052));
#28392=CARTESIAN_POINT('Ctrl Pts',(-4.55674969938714,-72.9338541062472,
26.935888782133));
#28393=CARTESIAN_POINT('Ctrl Pts',(-4.55145557742484,-72.931512042168,26.9365922725199));
#28394=CARTESIAN_POINT('Ctrl Pts',(-4.54583399063082,-72.9290251110787,
26.9373392768952));
#28395=CARTESIAN_POINT('Ctrl Pts',(-4.53957792038129,-72.9262559163629,
26.938164142488));
#28396=CARTESIAN_POINT('Ctrl Pts',(-4.53266052960038,-72.9231908648878,
26.9390654925595));
#28397=CARTESIAN_POINT('Ctrl Pts',(-4.52537764142081,-72.9199638638603,
26.9400144676846));
#28398=CARTESIAN_POINT('Ctrl Pts',(-4.51736195898021,-72.9164090127371,
26.941048150003));
#28399=CARTESIAN_POINT('Ctrl Pts',(-4.50863836855335,-72.9125349423682,
26.9421563442724));
#28400=CARTESIAN_POINT('Ctrl Pts',(-4.49929320103042,-72.9083848350362,
26.9433435000866));
#28401=CARTESIAN_POINT('Ctrl Pts',(-4.48913600582349,-72.9038685237529,
26.9446160351928));
#28402=CARTESIAN_POINT('Ctrl Pts',(-4.47825568517621,-72.8990223753879,
26.9459533685219));
#28403=CARTESIAN_POINT('Ctrl Pts',(-4.46619013276138,-72.8936483189604,
26.9474363822952));
#28404=CARTESIAN_POINT('Ctrl Pts',(-4.45323590238201,-72.8878688487667,
26.9489988385719));
#28405=CARTESIAN_POINT('Ctrl Pts',(-4.43957675807571,-72.881761889156,26.9506060319701));
#28406=CARTESIAN_POINT('Ctrl Pts',(-4.42279854385202,-72.874260403389,26.9525802284885));
#28407=CARTESIAN_POINT('Ctrl Pts',(-4.40495824690347,-72.8662653078568,
26.9546212264838));
#28408=CARTESIAN_POINT('Ctrl Pts',(-4.38647244881348,-72.8579574601868,
26.9566627807069));
#28409=CARTESIAN_POINT('Ctrl Pts',(-4.36758289127922,-72.8494681558146,
26.9587489257447));
#28410=CARTESIAN_POINT('Ctrl Pts',(-4.3480248947097,-72.8406547386207,26.9608347976216));
#28411=CARTESIAN_POINT('Ctrl Pts',(-4.32825338233612,-72.8317188036569,
26.9628611127856));
#28412=CARTESIAN_POINT('Ctrl Pts',(-4.3124762273609,-72.8245881589137,26.9644780598238));
#28413=CARTESIAN_POINT('Ctrl Pts',(-4.29656443351978,-72.8173801925865,
26.966057264346));
#28414=CARTESIAN_POINT('Ctrl Pts',(-4.28071697548282,-72.810184636013,26.9675781040822));
#28415=CARTESIAN_POINT('Ctrl Pts',(-4.26656300185773,-72.8037580079872,
26.9689364244806));
#28416=CARTESIAN_POINT('Ctrl Pts',(-4.25246083720482,-72.7973415389137,
26.9702482883927));
#28417=CARTESIAN_POINT('Ctrl Pts',(-4.23851320078447,-72.7909823721865,
26.9715057794914));
#28418=CARTESIAN_POINT('Ctrl Pts',(-4.22551505926242,-72.785056110088,26.9726776660227));
#28419=CARTESIAN_POINT('Ctrl Pts',(-4.21265145110638,-72.7791797850726,
26.9738024027896));
#28420=CARTESIAN_POINT('Ctrl Pts',(-4.19996403818309,-72.7733731934558,
26.974878671993));
#28421=CARTESIAN_POINT('Ctrl Pts',(-4.187915007338,-72.767858767314,26.9759007874477));
#28422=CARTESIAN_POINT('Ctrl Pts',(-4.17602513364819,-72.7624073601484,
26.9768792489206));
#28423=CARTESIAN_POINT('Ctrl Pts',(-4.16428725671022,-72.7570166654915,
26.9778167794621));
#28424=CARTESIAN_POINT('Ctrl Pts',(-4.15301887095358,-72.7518415876464,
26.9787168106905));
#28425=CARTESIAN_POINT('Ctrl Pts',(-4.14189076362031,-72.7467225623866,
26.9795791705336));
#28426=CARTESIAN_POINT('Ctrl Pts',(-4.13085286395148,-72.7416377006988,
26.9804091399343));
#28427=CARTESIAN_POINT('Ctrl Pts',(-4.11951589860725,-72.7364150675471,
26.9812615968885));
#28428=CARTESIAN_POINT('Ctrl Pts',(-4.10827476564544,-72.731228789118,26.9820799238327));
#28429=CARTESIAN_POINT('Ctrl Pts',(-4.09702051754996,-72.726030171066,26.9828723349526));
#28430=CARTESIAN_POINT('Ctrl Pts',(-4.08628526929532,-72.7210712919924,
26.9836282033163));
#28431=CARTESIAN_POINT('Ctrl Pts',(-4.07553030765988,-72.7160976402375,
26.9843609983902));
#28432=CARTESIAN_POINT('Ctrl Pts',(-4.06467325990052,-72.7110723521894,
26.9850752378722));
#28433=CARTESIAN_POINT('Ctrl Pts',(-4.05342869936957,-72.7058677001612,
26.9858149701888));
#28434=CARTESIAN_POINT('Ctrl Pts',(-4.04207482726141,-72.7006077368884,
26.9865347189675));
#28435=CARTESIAN_POINT('Ctrl Pts',(-4.0305704817495,-72.6952744058323,26.9872349869563));
#28436=CARTESIAN_POINT('Ctrl Pts',(-4.01826668589923,-72.6895704554035,
26.9879839173813));
#28437=CARTESIAN_POINT('Ctrl Pts',(-4.00579082229074,-72.683782595724,26.9887104787675));
#28438=CARTESIAN_POINT('Ctrl Pts',(-3.9931476618675,-72.6779139798043,26.989411499818));
#28439=CARTESIAN_POINT('Ctrl Pts',(-3.97973438237103,-72.671687895269,26.990155221401));
#28440=CARTESIAN_POINT('Ctrl Pts',(-3.96613313239916,-72.6653710564959,
26.9908700643548));
#28441=CARTESIAN_POINT('Ctrl Pts',(-3.95240663901933,-72.658993520968,26.9915498852838));
#28442=CARTESIAN_POINT('Ctrl Pts',(-3.93749262433767,-72.6520642451608,
26.9922885196193));
#28443=CARTESIAN_POINT('Ctrl Pts',(-3.92243124975649,-72.6450635337329,
26.9929856248137));
#28444=CARTESIAN_POINT('Ctrl Pts',(-3.90736223915333,-72.6380574390472,
26.993633202471));
#28445=CARTESIAN_POINT('Ctrl Pts',(-3.88988346046555,-72.6299309613573,
26.994384337821));
#28446=CARTESIAN_POINT('Ctrl Pts',(-3.87239532264419,-72.6217976615962,
26.9950684921256));
#28447=CARTESIAN_POINT('Ctrl Pts',(-3.85518253073393,-72.6137916939521,
26.9956775890504));
#28448=CARTESIAN_POINT('Ctrl Pts',(-3.83312496894388,-72.6035323399252,
26.9964581244292));
#28449=CARTESIAN_POINT('Ctrl Pts',(-3.81152482888409,-72.5934845725453,
26.9971144521718));
#28450=CARTESIAN_POINT('Ctrl Pts',(-3.79103926538539,-72.5839576125555,
26.9976485299609));
#28451=CARTESIAN_POINT('Ctrl Pts',(-3.77639774349918,-72.5771484665337,
26.9980302481225));
#28452=CARTESIAN_POINT('Ctrl Pts',(-3.76232753448869,-72.5706062766685,
26.9983500673601));
#28453=CARTESIAN_POINT('Ctrl Pts',(-3.74904725004508,-72.5644337382693,
26.9986154588061));
#28454=CARTESIAN_POINT('Ctrl Pts',(-3.73712649404653,-72.5588930945835,
26.9988536816157));
#28455=CARTESIAN_POINT('Ctrl Pts',(-3.72584290510903,-72.55365061639,26.999048201826));
#28456=CARTESIAN_POINT('Ctrl Pts',(-3.71532050420447,-72.5487644340811,
26.9992071337773));
#28457=CARTESIAN_POINT('Ctrl Pts',(-3.70549567633381,-72.5442021768012,
26.9993555294789));
#28458=CARTESIAN_POINT('Ctrl Pts',(-3.69633489253103,-72.5399507407298,
26.9994729902421));
#28459=CARTESIAN_POINT('Ctrl Pts',(-3.68790009473844,-72.5360390514937,
26.9995669997594));
#28460=CARTESIAN_POINT('Ctrl Pts',(-3.67988122234412,-72.5323202502132,
26.9996563736059));
#28461=CARTESIAN_POINT('Ctrl Pts',(-3.67251881961981,-72.5289086594291,
26.9997246070627));
#28462=CARTESIAN_POINT('Ctrl Pts',(-3.66582431552888,-72.5258095023081,
26.9997779400933));
#28463=CARTESIAN_POINT('Ctrl Pts',(-3.65939305483032,-72.5228322112168,
26.9998291759458));
#28464=CARTESIAN_POINT('Ctrl Pts',(-3.6535784467587,-72.5201433779329,26.9998666884134));
#28465=CARTESIAN_POINT('Ctrl Pts',(-3.64834700663704,-72.5177272092178,
26.9998952450266));
#28466=CARTESIAN_POINT('Ctrl Pts',(-3.64336360571696,-72.51542559874,26.99992244768));
#28467=CARTESIAN_POINT('Ctrl Pts',(-3.63890946442555,-72.5133714448824,
26.9999415292289));
#28468=CARTESIAN_POINT('Ctrl Pts',(-3.63491308271419,-72.5115312156491,
26.999955676367));
#28469=CARTESIAN_POINT('Ctrl Pts',(-3.63100696390056,-72.509732550119,26.9999695039757));
#28470=CARTESIAN_POINT('Ctrl Pts',(-3.62753836258856,-72.5081383474962,
26.9999786149847));
#28471=CARTESIAN_POINT('Ctrl Pts',(-3.62439655959128,-72.5066967962248,
26.999985050899));
#28472=CARTESIAN_POINT('Ctrl Pts',(-3.62135346789029,-72.5053005365884,
26.9999912846053));
#28473=CARTESIAN_POINT('Ctrl Pts',(-3.61861704716632,-72.50404752535,26.9999950010979));
#28474=CARTESIAN_POINT('Ctrl Pts',(-3.61604301879889,-72.502870335936,26.9999972537214));
#28475=CARTESIAN_POINT('Ctrl Pts',(-3.61387203465112,-72.5018774721475,
26.9999991536266));
#28476=CARTESIAN_POINT('Ctrl Pts',(-3.61181592875733,-72.500938245988,27.));
#28477=CARTESIAN_POINT('Ctrl Pts',(-3.60976192857619,-72.5,27.));
#28478=CARTESIAN_POINT('',(-4.20488096428809,-72.2245134174903,27.));
#28479=CARTESIAN_POINT('Ctrl Pts',(-4.59286900030108,-72.9498135639877,
26.9309674201926));
#28480=CARTESIAN_POINT('Ctrl Pts',(-4.97872124829708,-73.1202082891348,
26.87740515349));
#28481=CARTESIAN_POINT('Ctrl Pts',(-5.39943703784252,-73.2960271674307,
26.7866344447428));
#28482=CARTESIAN_POINT('Ctrl Pts',(-6.23069890002426,-73.6032059786734,
26.5355629374701));
#28483=CARTESIAN_POINT('Ctrl Pts',(-6.64131282637154,-73.7333042369875,
26.3751846606466));
#28484=CARTESIAN_POINT('Ctrl Pts',(-7.41892283648103,-73.9255858170934,
26.0143833640028));
#28485=CARTESIAN_POINT('Ctrl Pts',(-7.86775357562107,-74.000000000199,25.7653963103419));
#28486=CARTESIAN_POINT('Ctrl Pts',(-8.27069753274498,-74.,25.4999999988754));
#28487=CARTESIAN_POINT('Ctrl Pts',(-4.73222742226463,-72.6487711068476,
26.9529185755998));
#28488=CARTESIAN_POINT('Ctrl Pts',(-5.11803926821329,-72.8218353520906,
26.9133538137028));
#28489=CARTESIAN_POINT('Ctrl Pts',(-5.5378193485972,-73.0038698341822,26.8373083736856));
#28490=CARTESIAN_POINT('Ctrl Pts',(-6.36525494892567,-73.3302744149464,
26.613175065831));
#28491=CARTESIAN_POINT('Ctrl Pts',(-6.77293386456173,-73.473510370804,26.4648562596415));
#28492=CARTESIAN_POINT('Ctrl Pts',(-7.5432142505923,-73.6962982209631,26.123992425085));
#28493=CARTESIAN_POINT('Ctrl Pts',(-7.98659795783503,-73.7922248094884,
25.8845123595807));
#28494=CARTESIAN_POINT('Ctrl Pts',(-8.38308611702755,-73.8157835060006,
25.6245617146941));
#28495=CARTESIAN_POINT('Ctrl Pts',(-4.87158584422818,-72.3477286497075,
26.974869731007));
#28496=CARTESIAN_POINT('Ctrl Pts',(-5.25729552724842,-72.5236704313501,
26.9492448421667));
#28497=CARTESIAN_POINT('Ctrl Pts',(-5.67620378478722,-72.7117042159167,
26.8879934646398));
#28498=CARTESIAN_POINT('Ctrl Pts',(-6.49978013406627,-73.0574406580189,
26.6907209397854));
#28499=CARTESIAN_POINT('Ctrl Pts',(-6.90453460491355,-73.2137788863189,
26.5544817167923));
#28500=CARTESIAN_POINT('Ctrl Pts',(-7.66749336352552,-73.4670504132414,
26.2335669039408));
#28501=CARTESIAN_POINT('Ctrl Pts',(-8.10533935929029,-73.5847724306284,
26.0033054888075));
#28502=CARTESIAN_POINT('Ctrl Pts',(-8.49547470131012,-73.6315670120013,
25.7491234305128));
#28503=CARTESIAN_POINT('Ctrl Pts',(-5.01094426619173,-72.0466861925674,
26.9968208864141));
#28504=CARTESIAN_POINT('Ctrl Pts',(-5.39661354716464,-72.2252974943058,
26.9851935023795));
#28505=CARTESIAN_POINT('Ctrl Pts',(-5.8145860955419,-72.4195468826682,26.9386673935825));
#28506=CARTESIAN_POINT('Ctrl Pts',(-6.63433618296768,-72.7845090942918,
26.7683330681463));
#28507=CARTESIAN_POINT('Ctrl Pts',(-7.03615564310373,-72.9539850201353,
26.6441533157873));
#28508=CARTESIAN_POINT('Ctrl Pts',(-7.7917847776368,-73.2377628171111,26.3431759650231));
#28509=CARTESIAN_POINT('Ctrl Pts',(-8.22418374150425,-73.3769972399179,
26.1224215380463));
#28510=CARTESIAN_POINT('Ctrl Pts',(-8.60786328559268,-73.4473505180019,
25.8736851463315));
#28511=CARTESIAN_POINT('',(-8.60786328559223,-73.4473505180018,25.8736851463318));
#28512=CARTESIAN_POINT('Ctrl Pts',(-5.01094426619173,-72.0466861925674,
26.9968208864141));
#28513=CARTESIAN_POINT('Ctrl Pts',(-5.39661354716464,-72.2252974943058,
26.9851935023795));
#28514=CARTESIAN_POINT('Ctrl Pts',(-5.8145860955419,-72.4195468826682,26.9386673935825));
#28515=CARTESIAN_POINT('Ctrl Pts',(-6.63433618296768,-72.7845090942918,
26.7683330681463));
#28516=CARTESIAN_POINT('Ctrl Pts',(-7.03615564310373,-72.9539850201353,
26.6441533157873));
#28517=CARTESIAN_POINT('Ctrl Pts',(-7.7917847776368,-73.2377628171111,26.3431759650231));
#28518=CARTESIAN_POINT('Ctrl Pts',(-8.22418374150425,-73.3769972399179,
26.1224215380463));
#28519=CARTESIAN_POINT('Ctrl Pts',(-8.60786328559268,-73.4473505180019,
25.8736851463315));
#28520=CARTESIAN_POINT('',(-8.27069753304877,-74.,25.4999999993376));
#28521=CARTESIAN_POINT('',(-8.60786328559223,-73.4473505180018,25.8736851463318));
#28522=CARTESIAN_POINT('Ctrl Pts',(-8.27069753274498,-74.,25.4999999988754));
#28523=CARTESIAN_POINT('Ctrl Pts',(-7.86775357562107,-74.000000000199,25.7653963103419));
#28524=CARTESIAN_POINT('Ctrl Pts',(-7.41892283648103,-73.9255858170934,
26.0143833640028));
#28525=CARTESIAN_POINT('Ctrl Pts',(-6.64131282637154,-73.7333042369875,
26.3751846606466));
#28526=CARTESIAN_POINT('Ctrl Pts',(-6.23069890002426,-73.6032059786734,
26.5355629374701));
#28527=CARTESIAN_POINT('Ctrl Pts',(-5.39943703784252,-73.2960271674307,
26.7866344447428));
#28528=CARTESIAN_POINT('Ctrl Pts',(-4.97872124829708,-73.1202082891348,
26.87740515349));
#28529=CARTESIAN_POINT('Ctrl Pts',(-4.59286900030108,-72.9498135639877,
26.9309674201926));
#28530=CARTESIAN_POINT('Origin',(-4.79999999999999,-73.75,20.));
#28531=CARTESIAN_POINT('',(-10.3,-73.5,24.3301270189222));
#28532=CARTESIAN_POINT('',(-9.90714285714286,-74.,24.0208322318563));
#28533=CARTESIAN_POINT('',(-10.3,-73.5,24.3301270189222));
#28534=CARTESIAN_POINT('',(-8.82083223185632,-74.,25.1071428571429));
#28535=CARTESIAN_POINT('Origin',(-4.79999999999999,-74.,20.));
#28536=CARTESIAN_POINT('',(-9.13012701892219,-73.5,25.5));
#28537=CARTESIAN_POINT('',(-8.82083223185632,-74.,25.1071428571429));
#28538=CARTESIAN_POINT('Origin',(-4.79999999999999,-73.5,20.));
#28539=CARTESIAN_POINT('Ctrl Pts',(-8.2706975327445,-74.,25.4999999988757));
#28540=CARTESIAN_POINT('Ctrl Pts',(-8.46780983228826,-74.,25.3701733162485));
#28541=CARTESIAN_POINT('Ctrl Pts',(-8.65244115216739,-74.,25.2397164505804));
#28542=CARTESIAN_POINT('Ctrl Pts',(-8.82083223185632,-74.,25.1071428571429));
#28543=CARTESIAN_POINT('Ctrl Pts',(-8.38308611702708,-73.8157835060006,
25.6245617146944));
#28544=CARTESIAN_POINT('Ctrl Pts',(-8.57705715860084,-73.8272553216869,
25.4974516009823));
#28545=CARTESIAN_POINT('Ctrl Pts',(-8.75893190880213,-73.8333333333333,
25.3679979349617));
#28546=CARTESIAN_POINT('Ctrl Pts',(-8.92393049421161,-73.8333333333333,
25.2380952380952));
#28547=CARTESIAN_POINT('Ctrl Pts',(-8.49547470130966,-73.6315670120012,
25.7491234305131));
#28548=CARTESIAN_POINT('Ctrl Pts',(-8.68630448491342,-73.6545106433737,
25.6247298857161));
#28549=CARTESIAN_POINT('Ctrl Pts',(-8.86542266543686,-73.6666666666667,
25.496279419343));
#28550=CARTESIAN_POINT('Ctrl Pts',(-9.0270287565669,-73.6666666666667,25.3690476190476));
#28551=CARTESIAN_POINT('Ctrl Pts',(-8.60786328559223,-73.4473505180018,
25.8736851463318));
#28552=CARTESIAN_POINT('Ctrl Pts',(-8.795551811226,-73.4817659650606,25.7520081704499));
#28553=CARTESIAN_POINT('Ctrl Pts',(-8.97191342207159,-73.5,25.6245609037243));
#28554=CARTESIAN_POINT('Ctrl Pts',(-9.13012701892219,-73.5,25.5));
#28555=CARTESIAN_POINT('Ctrl Pts',(-8.82083223185632,-74.,25.1071428571429));
#28556=CARTESIAN_POINT('Ctrl Pts',(-8.65244115216739,-74.,25.2397164505804));
#28557=CARTESIAN_POINT('Ctrl Pts',(-8.46780983228826,-74.,25.3701733162485));
#28558=CARTESIAN_POINT('Ctrl Pts',(-8.2706975327445,-74.,25.4999999988757));
#28559=CARTESIAN_POINT('Ctrl Pts',(-8.60786328559223,-73.4473505180018,
25.8736851463318));
#28560=CARTESIAN_POINT('Ctrl Pts',(-8.795551811226,-73.4817659650606,25.7520081704499));
#28561=CARTESIAN_POINT('Ctrl Pts',(-8.97191342207159,-73.5,25.6245609037243));
#28562=CARTESIAN_POINT('Ctrl Pts',(-9.13012701892219,-73.5,25.5));
#28563=CARTESIAN_POINT('Ctrl Pts',(-10.299999999979,-74.,23.4706975310694));
#28564=CARTESIAN_POINT('Ctrl Pts',(-10.6578919709938,-74.000000000005,22.9273199449621));
#28565=CARTESIAN_POINT('Ctrl Pts',(-11.3040157101811,-73.7466600445013,
21.7070019367622));
#28566=CARTESIAN_POINT('Ctrl Pts',(-11.645906962903,-73.2204120541234,20.4056287461521));
#28567=CARTESIAN_POINT('Ctrl Pts',(-11.7309675556501,-72.9498131330638,
19.7928680244678));
#28568=CARTESIAN_POINT('Ctrl Pts',(-10.4245617157746,-73.8157835059031,
23.5830861153787));
#28569=CARTESIAN_POINT('Ctrl Pts',(-10.7749649472824,-73.7841592615321,
23.0483680049966));
#28570=CARTESIAN_POINT('Ctrl Pts',(-11.3929741147526,-73.4750024331891,
21.8418287216067));
#28571=CARTESIAN_POINT('Ctrl Pts',(-11.6900564874004,-72.9237209037276,
20.5448942447467));
#28572=CARTESIAN_POINT('Ctrl Pts',(-11.7529186757946,-72.648770667648,19.9322264436722));
#28573=CARTESIAN_POINT('Ctrl Pts',(-10.5491234315702,-73.6315670118063,
23.6954746996879));
#28574=CARTESIAN_POINT('Ctrl Pts',(-10.892037923571,-73.5683185230592,23.1694160650311));
#28575=CARTESIAN_POINT('Ctrl Pts',(-11.4819325193241,-73.203344821877,21.9766555064513));
#28576=CARTESIAN_POINT('Ctrl Pts',(-11.7342060118978,-72.6270297533319,
20.6841597433414));
#28577=CARTESIAN_POINT('Ctrl Pts',(-11.7748697959391,-72.3477282022321,
20.0715848628766));
#28578=CARTESIAN_POINT('Ctrl Pts',(-10.6736851473658,-73.4473505177094,
23.8078632839972));
#28579=CARTESIAN_POINT('Ctrl Pts',(-11.0091108998596,-73.3524777845862,
23.2904641250657));
#28580=CARTESIAN_POINT('Ctrl Pts',(-11.5708909238955,-72.9316872105648,
22.1114822912959));
#28581=CARTESIAN_POINT('Ctrl Pts',(-11.7783555363952,-72.3303386029362,
20.823425241936));
#28582=CARTESIAN_POINT('Ctrl Pts',(-11.7968209160836,-72.0466857368163,
20.210943282081));
#28583=CARTESIAN_POINT('',(-10.2999999999876,-74.,23.4706975310751));
#28584=CARTESIAN_POINT('Ctrl Pts',(-11.7309675556501,-72.9498131330638,
19.7928680244678));
#28585=CARTESIAN_POINT('Ctrl Pts',(-11.645906962903,-73.2204120541234,20.4056287461521));
#28586=CARTESIAN_POINT('Ctrl Pts',(-11.3040157101811,-73.7466600445013,
21.7070019367622));
#28587=CARTESIAN_POINT('Ctrl Pts',(-10.6578919709938,-74.000000000005,22.9273199449621));
#28588=CARTESIAN_POINT('Ctrl Pts',(-10.299999999979,-74.,23.4706975310694));
#28589=CARTESIAN_POINT('',(-10.6736851473658,-73.4473505177094,23.8078632839972));
#28590=CARTESIAN_POINT('',(-10.2999999999876,-74.,23.4706975310751));
#28591=CARTESIAN_POINT('Ctrl Pts',(-10.6736851473658,-73.4473505177094,
23.8078632839972));
#28592=CARTESIAN_POINT('Ctrl Pts',(-11.0091108998596,-73.3524777845862,
23.2904641250657));
#28593=CARTESIAN_POINT('Ctrl Pts',(-11.5708909238955,-72.9316872105648,
22.1114822912959));
#28594=CARTESIAN_POINT('Ctrl Pts',(-11.7783555363952,-72.3303386029362,
20.823425241936));
#28595=CARTESIAN_POINT('Ctrl Pts',(-11.7968209160836,-72.0466857368163,
20.210943282081));
#28596=CARTESIAN_POINT('Ctrl Pts',(-9.90714285714286,-74.,24.0208322318563));
#28597=CARTESIAN_POINT('Ctrl Pts',(-10.0446625272125,-74.,23.8461587910824));
#28598=CARTESIAN_POINT('Ctrl Pts',(-10.1730966676381,-74.,23.6633713879345));
#28599=CARTESIAN_POINT('Ctrl Pts',(-10.299999999979,-74.,23.4706975310694));
#28600=CARTESIAN_POINT('Ctrl Pts',(-10.0380952380952,-73.8333333333333,
24.1239304942116));
#28601=CARTESIAN_POINT('Ctrl Pts',(-10.1728443653613,-73.8333333333333,
23.9527761154313));
#28602=CARTESIAN_POINT('Ctrl Pts',(-10.3003137824798,-73.8269970069562,
23.7726894470159));
#28603=CARTESIAN_POINT('Ctrl Pts',(-10.4245617157746,-73.8157835059031,
23.5830861153787));
#28604=CARTESIAN_POINT('Ctrl Pts',(-10.1690476190476,-73.6666666666667,
24.2270287565669));
#28605=CARTESIAN_POINT('Ctrl Pts',(-10.3010262035101,-73.6666666666667,
24.0593934397802));
#28606=CARTESIAN_POINT('Ctrl Pts',(-10.4275308973216,-73.6539940139125,
23.8820075060973));
#28607=CARTESIAN_POINT('Ctrl Pts',(-10.5491234315702,-73.6315670118063,
23.6954746996879));
#28608=CARTESIAN_POINT('Ctrl Pts',(-10.3,-73.5,24.3301270189222));
#28609=CARTESIAN_POINT('Ctrl Pts',(-10.4292080416589,-73.5,24.1660107641291));
#28610=CARTESIAN_POINT('Ctrl Pts',(-10.5547480121633,-73.4809910208688,
23.9913255651787));
#28611=CARTESIAN_POINT('Ctrl Pts',(-10.6736851473658,-73.4473505177094,
23.8078632839972));
#28612=CARTESIAN_POINT('Ctrl Pts',(-10.299999999979,-74.,23.4706975310694));
#28613=CARTESIAN_POINT('Ctrl Pts',(-10.1730966676381,-74.,23.6633713879345));
#28614=CARTESIAN_POINT('Ctrl Pts',(-10.0446625272125,-74.,23.8461587910824));
#28615=CARTESIAN_POINT('Ctrl Pts',(-9.90714285714286,-74.,24.0208322318563));
#28616=CARTESIAN_POINT('Ctrl Pts',(-10.3,-73.5,24.3301270189222));
#28617=CARTESIAN_POINT('Ctrl Pts',(-10.4292080416589,-73.5,24.1660107641291));
#28618=CARTESIAN_POINT('Ctrl Pts',(-10.5547480121633,-73.4809910208688,
23.9913255651787));
#28619=CARTESIAN_POINT('Ctrl Pts',(-10.6736851473658,-73.4473505177094,
23.8078632839972));
#28620=CARTESIAN_POINT('Origin',(-10.3,-72.5,10.));
#28621=CARTESIAN_POINT('',(-10.3,-74.,10.));
#28622=CARTESIAN_POINT('',(-11.8,-72.5,10.));
#28623=CARTESIAN_POINT('Origin',(-11.8,-32.,20.));
#28624=CARTESIAN_POINT('',(-11.8,-32.,20.));
#28625=CARTESIAN_POINT('Origin',(-4.79999999999999,-32.,20.));
#28626=CARTESIAN_POINT('',(-4.8,-32.,27.));
#28627=CARTESIAN_POINT('Origin',(28.2,-73.75,-3.99999999999999));
#28628=CARTESIAN_POINT('',(28.2,-74.,-11.5));
#28629=CARTESIAN_POINT('',(28.2,-73.5,-11.));
#28630=CARTESIAN_POINT('',(35.7,-74.,-4.));
#28631=CARTESIAN_POINT('Origin',(28.2,-74.,-3.99999999999999));
#28632=CARTESIAN_POINT('',(35.7,-74.,-4.));
#28633=CARTESIAN_POINT('Origin',(21.7,-73.75,-11.25));
#28634=CARTESIAN_POINT('',(2.2,-74.,-11.5));
#28635=CARTESIAN_POINT('',(2.2,-73.5,-11.));
#28636=CARTESIAN_POINT('',(21.7,-74.,-11.5));
#28637=CARTESIAN_POINT('Origin',(2.2,-73.75,-4.));
#28638=CARTESIAN_POINT('',(-5.3,-74.,-4.));
#28639=CARTESIAN_POINT('',(-4.8,-73.5,-4.));
#28640=CARTESIAN_POINT('Origin',(2.2,-74.,-4.));
#28641=CARTESIAN_POINT('Origin',(-5.05,-73.75,-2.));
#28642=CARTESIAN_POINT('',(-5.3,-74.,4.));
#28643=CARTESIAN_POINT('',(-4.8,-73.5,4.));
#28644=CARTESIAN_POINT('',(-5.3,-74.,-2.));
#28645=CARTESIAN_POINT('Origin',(2.2,-73.75,4.));
#28646=CARTESIAN_POINT('',(2.2,-73.5,11.));
#28647=CARTESIAN_POINT('',(2.2,-74.,11.5));
#28648=CARTESIAN_POINT('',(2.2,-73.5,11.));
#28649=CARTESIAN_POINT('Origin',(2.2,-74.,4.));
#28650=CARTESIAN_POINT('Origin',(2.2,-73.5,4.));
#28651=CARTESIAN_POINT('Origin',(8.7,-73.75,11.25));
#28652=CARTESIAN_POINT('',(28.2,-73.5,11.));
#28653=CARTESIAN_POINT('',(28.2,-74.,11.5));
#28654=CARTESIAN_POINT('',(28.2,-73.5,11.));
#28655=CARTESIAN_POINT('',(8.7,-74.,11.5));
#28656=CARTESIAN_POINT('',(8.7,-73.5,11.));
#28657=CARTESIAN_POINT('Origin',(28.2,-73.75,3.99999999999999));
#28658=CARTESIAN_POINT('',(35.2,-73.5,4.));
#28659=CARTESIAN_POINT('',(35.7,-74.,4.));
#28660=CARTESIAN_POINT('',(35.2,-73.5,4.));
#28661=CARTESIAN_POINT('Origin',(28.2,-74.,3.99999999999999));
#28662=CARTESIAN_POINT('Origin',(28.2,-73.5,3.99999999999999));
#28663=CARTESIAN_POINT('Origin',(35.45,-73.75,2.));
#28664=CARTESIAN_POINT('',(35.7,-74.,2.));
#28665=CARTESIAN_POINT('',(35.2,-73.5,2.));
#28666=CARTESIAN_POINT('Origin',(15.2,-74.,0.));
#28667=CARTESIAN_POINT('',(39.2208322318563,-74.,-25.1071428571429));
#28668=CARTESIAN_POINT('Ctrl Pts',(39.2208322318563,-74.,-25.1071428571429));
#28669=CARTESIAN_POINT('Ctrl Pts',(39.0524411521674,-74.,-25.2397164505804));
#28670=CARTESIAN_POINT('Ctrl Pts',(38.8678098322883,-74.,-25.3701733162485));
#28671=CARTESIAN_POINT('Ctrl Pts',(38.6706975327445,-74.,-25.4999999988757));
#28672=CARTESIAN_POINT('',(40.3071428571429,-74.,-24.0208322318563));
#28673=CARTESIAN_POINT('Origin',(35.2,-74.,-20.));
#28674=CARTESIAN_POINT('',(40.6999999999876,-74.,-23.4706975310751));
#28675=CARTESIAN_POINT('Ctrl Pts',(40.699999999979,-74.,-23.4706975310694));
#28676=CARTESIAN_POINT('Ctrl Pts',(40.5730966676381,-74.,-23.6633713879345));
#28677=CARTESIAN_POINT('Ctrl Pts',(40.4446625272125,-74.,-23.8461587910824));
#28678=CARTESIAN_POINT('Ctrl Pts',(40.3071428571429,-74.,-24.0208322318563));
#28679=CARTESIAN_POINT('',(40.6999999999876,-74.,23.4706975310751));
#28680=CARTESIAN_POINT('',(40.7,-74.,-10.));
#28681=CARTESIAN_POINT('',(40.3071428571429,-74.,24.0208322318563));
#28682=CARTESIAN_POINT('Ctrl Pts',(40.3071428571429,-74.,24.0208322318563));
#28683=CARTESIAN_POINT('Ctrl Pts',(40.4446625272125,-74.,23.8461587910824));
#28684=CARTESIAN_POINT('Ctrl Pts',(40.5730966676381,-74.,23.6633713879345));
#28685=CARTESIAN_POINT('Ctrl Pts',(40.699999999979,-74.,23.4706975310694));
#28686=CARTESIAN_POINT('',(39.2208322318563,-74.,25.1071428571429));
#28687=CARTESIAN_POINT('Origin',(35.2,-74.,20.));
#28688=CARTESIAN_POINT('',(38.6706975330488,-74.,25.4999999993376));
#28689=CARTESIAN_POINT('Ctrl Pts',(38.6706975327445,-74.,25.4999999988757));
#28690=CARTESIAN_POINT('Ctrl Pts',(38.8678098322883,-74.,25.3701733162485));
#28691=CARTESIAN_POINT('Ctrl Pts',(39.0524411521674,-74.,25.2397164505804));
#28692=CARTESIAN_POINT('Ctrl Pts',(39.2208322318563,-74.,25.1071428571429));
#28693=CARTESIAN_POINT('',(25.2,-74.,25.5));
#28694=CARTESIAN_POINT('Ctrl Pts',(42.1309675556502,-72.9498131330638,-19.7928680244677));
#28695=CARTESIAN_POINT('Ctrl Pts',(42.131923849979,-72.9467709227376,-19.7859790576246));
#28696=CARTESIAN_POINT('Ctrl Pts',(42.133797063601,-72.9403541455888,-19.7715233813563));
#28697=CARTESIAN_POINT('Ctrl Pts',(42.1456478927983,-72.9035142121456,-19.6878036355088));
#28698=CARTESIAN_POINT('Ctrl Pts',(42.1734428705064,-72.7907445730559,-19.4364940183831));
#28699=CARTESIAN_POINT('Ctrl Pts',(42.1924901636104,-72.6655767127841,-19.1664431126415));
#28700=CARTESIAN_POINT('Ctrl Pts',(42.2001344080601,-72.5485934007217,-18.915145489479));
#28701=CARTESIAN_POINT('Ctrl Pts',(42.1998426464822,-72.5097904998462,-18.8311910013897));
#28702=CARTESIAN_POINT('Ctrl Pts',(42.2,-72.5031610690666,-18.8166823681909));
#28703=CARTESIAN_POINT('Ctrl Pts',(42.2,-72.5,-18.8097619285762));
#28704=CARTESIAN_POINT('Ctrl Pts',(42.1529186757946,-72.648770667648,-19.9322264436722));
#28705=CARTESIAN_POINT('Ctrl Pts',(42.1533741068936,-72.646492978889,-19.9271259487491));
#28706=CARTESIAN_POINT('Ctrl Pts',(42.1541647577967,-72.6424665483818,-19.9181031879452));
#28707=CARTESIAN_POINT('Ctrl Pts',(42.1623825078698,-72.6172309744667,-19.8602288521345));
#28708=CARTESIAN_POINT('Ctrl Pts',(42.1851067535948,-72.5287881205757,-19.662281685792));
#28709=CARTESIAN_POINT('Ctrl Pts',(42.1974831260006,-72.4421778837754,-19.4764677420227));
#28710=CARTESIAN_POINT('Ctrl Pts',(42.2015588908678,-72.3497072427885,-19.2786154621961));
#28711=CARTESIAN_POINT('Ctrl Pts',(42.1999951134572,-72.3228008493618,-19.2206366736043));
#28712=CARTESIAN_POINT('Ctrl Pts',(42.2,-72.3186768516068,-19.2116122804521));
#28713=CARTESIAN_POINT('Ctrl Pts',(42.2,-72.3163422783269,-19.2065079523841));
#28714=CARTESIAN_POINT('Ctrl Pts',(42.1748697959391,-72.3477282022321,-20.0715848628766));
#28715=CARTESIAN_POINT('Ctrl Pts',(42.1750197265735,-72.3462456838324,-20.0683082748074));
#28716=CARTESIAN_POINT('Ctrl Pts',(42.1755923536803,-72.3423623098006,-20.0597599196363));
#28717=CARTESIAN_POINT('Ctrl Pts',(42.1789294016785,-72.3223172427598,-20.0158885701159));
#28718=CARTESIAN_POINT('Ctrl Pts',(42.1857191167759,-72.2729880555877,-19.9084435042539));
#28719=CARTESIAN_POINT('Ctrl Pts',(42.1947085871064,-72.2076838276853,-19.7662744561243));
#28720=CARTESIAN_POINT('Ctrl Pts',(42.1983926835278,-72.1582937197183,-19.658974397133));
#28721=CARTESIAN_POINT('Ctrl Pts',(42.1997583650979,-72.138122537015,-19.6151072161929));
#28722=CARTESIAN_POINT('Ctrl Pts',(42.2,-72.134192634147,-19.6065421927134));
#28723=CARTESIAN_POINT('Ctrl Pts',(42.2,-72.1326845566538,-19.6032539761921));
#28724=CARTESIAN_POINT('Ctrl Pts',(42.1968209160836,-72.0466857368163,-20.2109432820811));
#28725=CARTESIAN_POINT('Ctrl Pts',(42.1968652729023,-72.0460043569063,-20.2094720016796));
#28726=CARTESIAN_POINT('Ctrl Pts',(42.1969519717285,-72.0445740919435,-20.2063835241584));
#28727=CARTESIAN_POINT('Ctrl Pts',(42.1975052667492,-72.0362656373519,-20.1884440303172));
#28728=CARTESIAN_POINT('Ctrl Pts',(42.1987929410797,-72.0112736650882,-20.1344713791154));
#28729=CARTESIAN_POINT('Ctrl Pts',(42.1996557903764,-71.9844299252291,-20.0764806253147));
#28730=CARTESIAN_POINT('Ctrl Pts',(42.2000060026571,-71.9594531297301,-20.0225217576406));
#28731=CARTESIAN_POINT('Ctrl Pts',(42.199992764164,-71.9511381123642,-20.0045600356903));
#28732=CARTESIAN_POINT('Ctrl Pts',(42.2,-71.9497084166872,-20.0014721049746));
#28733=CARTESIAN_POINT('Ctrl Pts',(42.2,-71.9490268349807,-20.));
#28734=CARTESIAN_POINT('',(42.1309675556502,-72.9498131330638,-19.7928680244677));
#28735=CARTESIAN_POINT('Ctrl Pts',(42.2,-72.5,-18.8097619285762));
#28736=CARTESIAN_POINT('Ctrl Pts',(42.2,-72.501104434069,-18.8121798350255));
#28737=CARTESIAN_POINT('Ctrl Pts',(42.199998844824,-72.5022107400032,-18.8146017627203));
#28738=CARTESIAN_POINT('Ctrl Pts',(42.1999961395225,-72.5034031482093,-18.8172080904455));
#28739=CARTESIAN_POINT('Ctrl Pts',(42.1999933680139,-72.5046247382961,-18.8198782029923));
#28740=CARTESIAN_POINT('Ctrl Pts',(42.1999889720745,-72.5059366396841,-18.8227417275941));
#28741=CARTESIAN_POINT('Ctrl Pts',(42.1999817153247,-72.5074063278034,-18.8259430216939));
#28742=CARTESIAN_POINT('Ctrl Pts',(42.1999742566232,-72.5089169166043,-18.8292334061994));
#28743=CARTESIAN_POINT('Ctrl Pts',(42.1999637834255,-72.5105941315298,-18.83288047915));
#28744=CARTESIAN_POINT('Ctrl Pts',(42.1999480152244,-72.5124880592726,-18.8369912426304));
#28745=CARTESIAN_POINT('Ctrl Pts',(42.199931738317,-72.5144430880226,-18.8412346256315));
#28746=CARTESIAN_POINT('Ctrl Pts',(42.1999098218899,-72.5166289622411,-18.8459719331802));
#28747=CARTESIAN_POINT('Ctrl Pts',(42.1998786784034,-72.519077475485,-18.8512709182691));
#28748=CARTESIAN_POINT('Ctrl Pts',(42.1998456108804,-72.521677257239,-18.8568972732759));
#28749=CARTESIAN_POINT('Ctrl Pts',(42.1998021319534,-72.5245731226336,-18.8631568226207));
#28750=CARTESIAN_POINT('Ctrl Pts',(42.1997427762118,-72.5277777824962,-18.8700764316876));
#28751=CARTESIAN_POINT('Ctrl Pts',(42.1996802900758,-72.5311514546458,-18.8773609777533));
#28752=CARTESIAN_POINT('Ctrl Pts',(42.1996001669454,-72.5348672363335,-18.885376785242));
#28753=CARTESIAN_POINT('Ctrl Pts',(42.1994951564366,-72.5389136971141,-18.8940991505866));
#28754=CARTESIAN_POINT('Ctrl Pts',(42.1993826824823,-72.5432477533007,-18.9034414434035));
#28755=CARTESIAN_POINT('Ctrl Pts',(42.1992415706987,-72.5479610044146,-18.9135939447025));
#28756=CARTESIAN_POINT('Ctrl Pts',(42.1990629471554,-72.5530120784886,-18.9244681723167));
#28757=CARTESIAN_POINT('Ctrl Pts',(42.1988649429093,-72.5586111954687,-18.9365222565747));
#28758=CARTESIAN_POINT('Ctrl Pts',(42.1986206702861,-72.5646251589739,-18.949462607627));
#28759=CARTESIAN_POINT('Ctrl Pts',(42.1983202304374,-72.5709682116296,-18.9631064122639));
#28760=CARTESIAN_POINT('Ctrl Pts',(42.1979524431967,-72.5787331397672,-18.9798086482816));
#28761=CARTESIAN_POINT('Ctrl Pts',(42.1974999722516,-72.5869905301771,-18.9975635488969));
#28762=CARTESIAN_POINT('Ctrl Pts',(42.1969538016202,-72.5955474532101,-19.0159607182467));
#28763=CARTESIAN_POINT('Ctrl Pts',(42.1963926885024,-72.6043384820296,-19.0348612091509));
#28764=CARTESIAN_POINT('Ctrl Pts',(42.1957325786725,-72.6134430509651,-19.0544340658138));
#28765=CARTESIAN_POINT('Ctrl Pts',(42.1949775407195,-72.6226464542665,-19.0742232187686));
#28766=CARTESIAN_POINT('Ctrl Pts',(42.1943746852057,-72.6299948562963,-19.0900237489613));
#28767=CARTESIAN_POINT('Ctrl Pts',(42.1937117025218,-72.6374056335292,-19.1059608261784));
#28768=CARTESIAN_POINT('Ctrl Pts',(42.1929961401609,-72.6447844102958,-19.121834298351));
#28769=CARTESIAN_POINT('Ctrl Pts',(42.192357485478,-72.6513701260813,-19.13600171113));
#28770=CARTESIAN_POINT('Ctrl Pts',(42.1916771251311,-72.6579301278482,-19.1501179668197));
#28771=CARTESIAN_POINT('Ctrl Pts',(42.1909619574118,-72.6644154541118,-19.164079711081));
#28772=CARTESIAN_POINT('Ctrl Pts',(42.1902956522372,-72.6704576821534,-19.1770875443427));
#28773=CARTESIAN_POINT('Ctrl Pts',(42.1895992563686,-72.67643494612,-19.1899609298698));
#28774=CARTESIAN_POINT('Ctrl Pts',(42.1888777417672,-72.6823268221358,-19.2026576733762));
#28775=CARTESIAN_POINT('Ctrl Pts',(42.188192629382,-72.687921438271,-19.2147138344182));
#28776=CARTESIAN_POINT('Ctrl Pts',(42.1874849648869,-72.693438960502,-19.2266104811067));
#28777=CARTESIAN_POINT('Ctrl Pts',(42.1867569121392,-72.6988815833764,-19.2383542485828));
#28778=CARTESIAN_POINT('Ctrl Pts',(42.1860580430634,-72.7041060411239,-19.2496272723423));
#28779=CARTESIAN_POINT('Ctrl Pts',(42.1853404669399,-72.7092614026533,-19.2607592299263));
#28780=CARTESIAN_POINT('Ctrl Pts',(42.1846028726667,-72.7143695651666,-19.2717996399122));
#28781=CARTESIAN_POINT('Ctrl Pts',(42.183851133165,-72.7195756895659,-19.2830517775752));
#28782=CARTESIAN_POINT('Ctrl Pts',(42.1830787256542,-72.724732519747,-19.2942082079408));
#28783=CARTESIAN_POINT('Ctrl Pts',(42.1822792532141,-72.729887397417,-19.3053745694477));
#28784=CARTESIAN_POINT('Ctrl Pts',(42.1815108442835,-72.7348419822639,-19.3161070618675));
#28785=CARTESIAN_POINT('Ctrl Pts',(42.1807168472024,-72.7397983610905,-19.3268566425136));
#28786=CARTESIAN_POINT('Ctrl Pts',(42.1798905612537,-72.7447936410782,-19.3377066031676));
#28787=CARTESIAN_POINT('Ctrl Pts',(42.1790348821558,-72.749966616221,-19.3489425252583));
#28788=CARTESIAN_POINT('Ctrl Pts',(42.1781445235793,-72.7551812136774,-19.3602859041663));
#28789=CARTESIAN_POINT('Ctrl Pts',(42.1772145611532,-72.7604556398254,-19.3717788059764));
#28790=CARTESIAN_POINT('Ctrl Pts',(42.1762202119558,-72.7660952455344,-19.3840674290118));
#28791=CARTESIAN_POINT('Ctrl Pts',(42.175180506677,-72.7718032174315,-19.3965269512495));
#28792=CARTESIAN_POINT('Ctrl Pts',(42.1740933204494,-72.7775768048783,-19.409153596826));
#28793=CARTESIAN_POINT('Ctrl Pts',(42.1729402752533,-72.7837001415259,-19.4225451323847));
#28794=CARTESIAN_POINT('Ctrl Pts',(42.1717337402546,-72.7898971149343,-19.4361243256636));
#28795=CARTESIAN_POINT('Ctrl Pts',(42.1704767177069,-72.7961388570958,-19.4498295830908));
#28796=CARTESIAN_POINT('Ctrl Pts',(42.1691117732258,-72.8029164853346,-19.4647115082577));
#28797=CARTESIAN_POINT('Ctrl Pts',(42.1676871916453,-72.8097466432141,-19.4797415851259));
#28798=CARTESIAN_POINT('Ctrl Pts',(42.1662147821111,-72.8165662848741,-19.4947816596442));
#28799=CARTESIAN_POINT('Ctrl Pts',(42.1645116079787,-72.8244547404951,-19.5121789022399));
#28800=CARTESIAN_POINT('Ctrl Pts',(42.1627442453548,-72.832328637204,-19.5295886154484));
#28801=CARTESIAN_POINT('Ctrl Pts',(42.1609440847193,-72.8400623197647,-19.5467306475705));
#28802=CARTESIAN_POINT('Ctrl Pts',(42.1585963565592,-72.8501484109563,-19.5690868921973));
#28803=CARTESIAN_POINT('Ctrl Pts',(42.1561926064094,-72.8599933687502,-19.5909825486671));
#28804=CARTESIAN_POINT('Ctrl Pts',(42.153829461459,-72.8692964892791,-19.611733851028));
#28805=CARTESIAN_POINT('Ctrl Pts',(42.1521606565976,-72.8758661636286,-19.626387998356));
#28806=CARTESIAN_POINT('Ctrl Pts',(42.1505129132781,-72.8821649104918,-19.6404694774991));
#28807=CARTESIAN_POINT('Ctrl Pts',(42.1489236489795,-72.8880982600165,-19.6537587709998));
#28808=CARTESIAN_POINT('Ctrl Pts',(42.1474976601363,-72.8934220379641,-19.6656827689679));
#28809=CARTESIAN_POINT('Ctrl Pts',(42.146118990168,-72.8984513774561,-19.6769682936815));
#28810=CARTESIAN_POINT('Ctrl Pts',(42.1448124401236,-72.9031339887235,-19.6874909539755));
#28811=CARTESIAN_POINT('Ctrl Pts',(42.1435926877886,-72.9075055212581,-19.6973145650335));
#28812=CARTESIAN_POINT('Ctrl Pts',(42.1424359361706,-72.9115747003091,-19.7064728666792));
#28813=CARTESIAN_POINT('Ctrl Pts',(42.1413577511395,-72.915316545818,-19.7149037671802));
#28814=CARTESIAN_POINT('Ctrl Pts',(42.1403328121502,-72.9188736007235,-19.7229183086448));
#28815=CARTESIAN_POINT('Ctrl Pts',(42.1393789657513,-72.9221347341472,-19.7302752031998));
#28816=CARTESIAN_POINT('Ctrl Pts',(42.1385035999543,-72.9250969217939,-19.7369630176399));
#28817=CARTESIAN_POINT('Ctrl Pts',(42.1376626969175,-72.9279424894365,-19.7433875358139));
#28818=CARTESIAN_POINT('Ctrl Pts',(42.1368942766262,-72.9305120885607,-19.7491943710542));
#28819=CARTESIAN_POINT('Ctrl Pts',(42.1361981280593,-72.9328220615438,-19.7544171202231));
#28820=CARTESIAN_POINT('Ctrl Pts',(42.1355350110767,-72.9350224285159,-19.7593920549341));
#28821=CARTESIAN_POINT('Ctrl Pts',(42.1349374860318,-72.9369871912694,-19.7638369366521));
#28822=CARTESIAN_POINT('Ctrl Pts',(42.1343986079509,-72.9387489413189,-19.7678234681457));
#28823=CARTESIAN_POINT('Ctrl Pts',(42.13387191165,-72.940470865567,-19.7717198808326));
#28824=CARTESIAN_POINT('Ctrl Pts',(42.1334012661809,-72.9419987635743,-19.7751782288515));
#28825=CARTESIAN_POINT('Ctrl Pts',(42.1329732356419,-72.9433821218023,-19.7783095280656));
#28826=CARTESIAN_POINT('Ctrl Pts',(42.1325586563635,-72.9447220067026,-19.7813424232698));
#28827=CARTESIAN_POINT('Ctrl Pts',(42.1321840603972,-72.9459262548977,-19.784068416823));
#28828=CARTESIAN_POINT('Ctrl Pts',(42.1318304518762,-72.9470587848148,-19.7866321657247));
#28829=CARTESIAN_POINT('Ctrl Pts',(42.1315331756714,-72.9480108947768,-19.7887874914539));
#28830=CARTESIAN_POINT('Ctrl Pts',(42.1312506313311,-72.948912598852,-19.7908287998052));
#28831=CARTESIAN_POINT('Ctrl Pts',(42.1309675556502,-72.9498131330638,-19.7928680244677));
#28832=CARTESIAN_POINT('Ctrl Pts',(42.1968209160836,-72.0466857368163,-20.2109432820811));
#28833=CARTESIAN_POINT('Ctrl Pts',(42.1748697959391,-72.3477282022321,-20.0715848628766));
#28834=CARTESIAN_POINT('Ctrl Pts',(42.1529186757946,-72.648770667648,-19.9322264436722));
#28835=CARTESIAN_POINT('Ctrl Pts',(42.1309675556502,-72.9498131330638,-19.7928680244677));
#28836=CARTESIAN_POINT('Ctrl Pts',(35.4109442661894,-72.0466861925664,-26.9968208864142));
#28837=CARTESIAN_POINT('Ctrl Pts',(35.4094729764645,-72.0460048083184,-26.9968652437211));
#28838=CARTESIAN_POINT('Ctrl Pts',(35.4063844798888,-72.044574534468,-26.9969519434978));
#28839=CARTESIAN_POINT('Ctrl Pts',(35.3884448933592,-72.0362660370501,-26.9975052438987));
#28840=CARTESIAN_POINT('Ctrl Pts',(35.3344720145561,-72.0112739574878,-26.9987929295366));
#28841=CARTESIAN_POINT('Ctrl Pts',(35.2764810198642,-71.9844300964231,-26.9996557867445));
#28842=CARTESIAN_POINT('Ctrl Pts',(35.2225218784051,-71.9594531763374,-27.0000060027141));
#28843=CARTESIAN_POINT('Ctrl Pts',(35.2045600608895,-71.9511381208737,-26.9999927640876));
#28844=CARTESIAN_POINT('Ctrl Pts',(35.2014721131251,-71.9497084193948,-27.));
#28845=CARTESIAN_POINT('Ctrl Pts',(35.2,-71.9490268349807,-27.));
#28846=CARTESIAN_POINT('Ctrl Pts',(35.2715858442274,-72.3477286497072,-26.9748697310069));
#28847=CARTESIAN_POINT('Ctrl Pts',(35.2683092255771,-72.3462461176061,-26.9750196643681));
#28848=CARTESIAN_POINT('Ctrl Pts',(35.2597589197381,-72.342362724116,-26.9755113943378));
#28849=CARTESIAN_POINT('Ctrl Pts',(35.2159130361133,-72.3223176226921,-26.9782700800717));
#28850=CARTESIAN_POINT('Ctrl Pts',(35.1085728978907,-72.2729884298032,-26.9845159160213));
#28851=CARTESIAN_POINT('Ctrl Pts',(34.9663896521622,-72.2076842086041,-26.9930983031639));
#28852=CARTESIAN_POINT('Ctrl Pts',(34.8590309097738,-72.1582939925205,-26.9980896019632));
#28853=CARTESIAN_POINT('Ctrl Pts',(34.8151119751847,-72.1381226464778,-26.99978388301));
#28854=CARTESIAN_POINT('Ctrl Pts',(34.8065421980393,-72.1341926745702,-27.));
#28855=CARTESIAN_POINT('Ctrl Pts',(34.8032539761921,-72.1326845566538,-27.));
#28856=CARTESIAN_POINT('Ctrl Pts',(35.1322274222654,-72.6487711068479,-26.9529185755996));
#28857=CARTESIAN_POINT('Ctrl Pts',(35.1271268758826,-72.6464933955941,-26.9533740167507));
#28858=CARTESIAN_POINT('Ctrl Pts',(35.1181040099963,-72.6425801185888,-26.954490007591));
#28859=CARTESIAN_POINT('Ctrl Pts',(35.0602294418299,-72.6159498143769,-26.9622965659357));
#28860=CARTESIAN_POINT('Ctrl Pts',(34.8622824530211,-72.5231676294432,-26.9782300245881));
#28861=CARTESIAN_POINT('Ctrl Pts',(34.6764682420516,-72.438402280726,-26.9937530473512));
#28862=CARTESIAN_POINT('Ctrl Pts',(34.4786155584546,-72.3480981199775,-26.9979624748782));
#28863=CARTESIAN_POINT('Ctrl Pts',(34.4206366861374,-72.322674383005,-26.9994067438287));
#28864=CARTESIAN_POINT('Ctrl Pts',(34.4116122829534,-72.3186769297456,-27.));
#28865=CARTESIAN_POINT('Ctrl Pts',(34.4065079523841,-72.3163422783269,-27.));
#28866=CARTESIAN_POINT('Ctrl Pts',(34.9928690003034,-72.9498135639887,-26.9309674201923));
#28867=CARTESIAN_POINT('Ctrl Pts',(34.9859799608414,-72.9467713218047,-26.9319237255421));
#28868=CARTESIAN_POINT('Ctrl Pts',(34.9715241428247,-72.9403544842611,-26.9337969592289));
#28869=CARTESIAN_POINT('Ctrl Pts',(34.8878040852748,-72.9035143512801,-26.9456478606198));
#28870=CARTESIAN_POINT('Ctrl Pts',(34.6364946325283,-72.7907448177968,-26.9734427948335));
#28871=CARTESIAN_POINT('Ctrl Pts',(34.3664435092558,-72.6655780479714,-26.9924899951682));
#28872=CARTESIAN_POINT('Ctrl Pts',(34.1151455412382,-72.5485944343277,-27.0001343924598));
#28873=CARTESIAN_POINT('Ctrl Pts',(34.0311910031954,-72.5097908429465,-26.9998426436926));
#28874=CARTESIAN_POINT('Ctrl Pts',(34.0166823678675,-72.503161184921,-27.));
#28875=CARTESIAN_POINT('Ctrl Pts',(34.0097619285762,-72.5,-27.));
#28876=CARTESIAN_POINT('Ctrl Pts',(34.9928690003034,-72.9498135639887,-26.9309674201923));
#28877=CARTESIAN_POINT('Ctrl Pts',(35.1322274222654,-72.6487711068479,-26.9529185755996));
#28878=CARTESIAN_POINT('Ctrl Pts',(35.2715858442274,-72.3477286497072,-26.9748697310069));
#28879=CARTESIAN_POINT('Ctrl Pts',(35.4109442661894,-72.0466861925664,-26.9968208864142));
#28880=CARTESIAN_POINT('Ctrl Pts',(34.9928690003034,-72.9498135639887,-26.9309674201923));
#28881=CARTESIAN_POINT('Ctrl Pts',(35.3787212463313,-73.1202082882644,-26.8774051537635));
#28882=CARTESIAN_POINT('Ctrl Pts',(35.7977539931684,-73.2955896700455,-26.7874092748223));
#28883=CARTESIAN_POINT('Ctrl Pts',(36.7538439760921,-73.6459407607355,-26.4950027398036));
#28884=CARTESIAN_POINT('Ctrl Pts',(37.5431082034452,-73.8929551961393,-26.1757552250324));
#28885=CARTESIAN_POINT('Ctrl Pts',(38.3641779127485,-74.0000000001514,-25.7018870729982));
#28886=CARTESIAN_POINT('Ctrl Pts',(38.670697532745,-74.,-25.4999999988754));
#28887=CARTESIAN_POINT('Ctrl Pts',(35.1322274222654,-72.6487711068479,-26.9529185755996));
#28888=CARTESIAN_POINT('Ctrl Pts',(35.5179816685701,-72.8220656430667,-26.9134786970919));
#28889=CARTESIAN_POINT('Ctrl Pts',(35.9362199946512,-73.003097605608,-26.8379018493463));
#28890=CARTESIAN_POINT('Ctrl Pts',(36.8877441571632,-73.376153426664,-26.5765090318869));
#28891=CARTESIAN_POINT('Ctrl Pts',(37.6709975247959,-73.6498315266744,-26.2802660100171));
#28892=CARTESIAN_POINT('Ctrl Pts',(38.4815957329272,-73.7974150709988,-25.8221481156266));
#28893=CARTESIAN_POINT('Ctrl Pts',(38.7830861170276,-73.8157835060006,-25.6245617146941));
#28894=CARTESIAN_POINT('Ctrl Pts',(35.2715858442274,-72.3477286497072,-26.9748697310069));
#28895=CARTESIAN_POINT('Ctrl Pts',(35.6573531268961,-72.5234401404136,-26.9491199589918));
#28896=CARTESIAN_POINT('Ctrl Pts',(36.0744840326391,-72.7114040323017,-26.888810351696));
#28897=CARTESIAN_POINT('Ctrl Pts',(37.021572601592,-73.1065740407313,-26.6577720692435));
#28898=CARTESIAN_POINT('Ctrl Pts',(37.7990763569512,-73.4059683812817,-26.3844509574549));
#28899=CARTESIAN_POINT('Ctrl Pts',(38.5985802916715,-73.5964176820098,-25.9426379705939));
#28900=CARTESIAN_POINT('Ctrl Pts',(38.8954747013101,-73.6315670120013,-25.7491234305128));
#28901=CARTESIAN_POINT('Ctrl Pts',(35.4109442661894,-72.0466861925664,-26.9968208864142));
#28902=CARTESIAN_POINT('Ctrl Pts',(35.7966135491349,-72.2252974952159,-26.9851935023203));
#28903=CARTESIAN_POINT('Ctrl Pts',(36.2129500341219,-72.4189119678641,-26.93930292622));
#28904=CARTESIAN_POINT('Ctrl Pts',(37.155472782663,-72.8367867066598,-26.7392783613268));
#28905=CARTESIAN_POINT('Ctrl Pts',(37.926965678302,-73.1628447118167,-26.4889617424396));
#28906=CARTESIAN_POINT('Ctrl Pts',(38.7159981118503,-73.3938327528572,-26.0628990132224));
#28907=CARTESIAN_POINT('Ctrl Pts',(39.0078632855927,-73.4473505180019,-25.8736851463315));
#28908=CARTESIAN_POINT('',(39.0078632855922,-73.4473505180018,-25.8736851463318));
#28909=CARTESIAN_POINT('Origin',(35.2,-73.75,-20.));
#28910=CARTESIAN_POINT('',(40.7,-73.5,-24.3301270189222));
#28911=CARTESIAN_POINT('',(39.2208322318563,-74.,-25.1071428571429));
#28912=CARTESIAN_POINT('Ctrl Pts',(38.6706975327445,-74.,-25.4999999988757));
#28913=CARTESIAN_POINT('Ctrl Pts',(38.8678098322883,-74.,-25.3701733162485));
#28914=CARTESIAN_POINT('Ctrl Pts',(39.0524411521674,-74.,-25.2397164505804));
#28915=CARTESIAN_POINT('Ctrl Pts',(39.2208322318563,-74.,-25.1071428571429));
#28916=CARTESIAN_POINT('Ctrl Pts',(38.7830861170271,-73.8157835060006,-25.6245617146944));
#28917=CARTESIAN_POINT('Ctrl Pts',(38.9770571586009,-73.8272553216869,-25.4974516009823));
#28918=CARTESIAN_POINT('Ctrl Pts',(39.1589319088021,-73.8333333333333,-25.3679979349617));
#28919=CARTESIAN_POINT('Ctrl Pts',(39.3239304942116,-73.8333333333333,-25.2380952380952));
#28920=CARTESIAN_POINT('Ctrl Pts',(38.8954747013097,-73.6315670120012,-25.7491234305131));
#28921=CARTESIAN_POINT('Ctrl Pts',(39.0863044849134,-73.6545106433737,-25.6247298857161));
#28922=CARTESIAN_POINT('Ctrl Pts',(39.2654226654369,-73.6666666666667,-25.496279419343));
#28923=CARTESIAN_POINT('Ctrl Pts',(39.4270287565669,-73.6666666666667,-25.3690476190476));
#28924=CARTESIAN_POINT('Ctrl Pts',(39.0078632855922,-73.4473505180018,-25.8736851463318));
#28925=CARTESIAN_POINT('Ctrl Pts',(39.195551811226,-73.4817659650606,-25.7520081704499));
#28926=CARTESIAN_POINT('Ctrl Pts',(39.3719134220716,-73.5,-25.6245609037243));
#28927=CARTESIAN_POINT('Ctrl Pts',(39.5301270189222,-73.5,-25.5));
#28928=CARTESIAN_POINT('Ctrl Pts',(40.699999999979,-74.,-23.4706975310694));
#28929=CARTESIAN_POINT('Ctrl Pts',(41.0578919709938,-74.000000000005,-22.9273199449621));
#28930=CARTESIAN_POINT('Ctrl Pts',(41.7040084948481,-73.7466609117147,-21.7069991633697));
#28931=CARTESIAN_POINT('Ctrl Pts',(42.0459069628923,-73.2204120541575,-20.4056287462293));
#28932=CARTESIAN_POINT('Ctrl Pts',(42.1309675556502,-72.9498131330637,-19.7928680244677));
#28933=CARTESIAN_POINT('Ctrl Pts',(40.8245617157746,-73.8157835059031,-23.5830861153787));
#28934=CARTESIAN_POINT('Ctrl Pts',(41.1749649472824,-73.7841592615321,-23.0483680049966));
#28935=CARTESIAN_POINT('Ctrl Pts',(41.7929663852314,-73.4750040339006,-21.8418257930973));
#28936=CARTESIAN_POINT('Ctrl Pts',(42.090056487394,-72.9237209037385,-20.5448942447724));
#28937=CARTESIAN_POINT('Ctrl Pts',(42.1529186757946,-72.648770667648,-19.9322264436722));
#28938=CARTESIAN_POINT('Ctrl Pts',(40.9491234315702,-73.6315670118063,-23.695474699688));
#28939=CARTESIAN_POINT('Ctrl Pts',(41.292037923571,-73.5683185230592,-23.1694160650312));
#28940=CARTESIAN_POINT('Ctrl Pts',(41.8819242756147,-73.2033471560866,-21.9766524228248));
#28941=CARTESIAN_POINT('Ctrl Pts',(42.1342060118958,-72.6270297533195,-20.6841597433155));
#28942=CARTESIAN_POINT('Ctrl Pts',(42.1748697959391,-72.3477282022321,-20.0715848628766));
#28943=CARTESIAN_POINT('Ctrl Pts',(41.0736851473658,-73.4473505177094,-23.8078632839972));
#28944=CARTESIAN_POINT('Ctrl Pts',(41.4091108998595,-73.3524777845863,-23.2904641250657));
#28945=CARTESIAN_POINT('Ctrl Pts',(41.9708821659981,-72.9316902782726,-22.1114790525524));
#28946=CARTESIAN_POINT('Ctrl Pts',(42.1783555363975,-72.3303386029005,-20.8234252418586));
#28947=CARTESIAN_POINT('Ctrl Pts',(42.1968209160836,-72.0466857368163,-20.2109432820811));
#28948=CARTESIAN_POINT('Ctrl Pts',(42.1309675556502,-72.9498131330637,-19.7928680244677));
#28949=CARTESIAN_POINT('Ctrl Pts',(42.0459069628923,-73.2204120541575,-20.4056287462293));
#28950=CARTESIAN_POINT('Ctrl Pts',(41.7040084948481,-73.7466609117147,-21.7069991633697));
#28951=CARTESIAN_POINT('Ctrl Pts',(41.0578919709938,-74.000000000005,-22.9273199449621));
#28952=CARTESIAN_POINT('Ctrl Pts',(40.699999999979,-74.,-23.4706975310694));
#28953=CARTESIAN_POINT('',(40.6999999999876,-74.,-23.4706975310751));
#28954=CARTESIAN_POINT('Ctrl Pts',(40.3071428571429,-74.,-24.0208322318563));
#28955=CARTESIAN_POINT('Ctrl Pts',(40.4446625272125,-74.,-23.8461587910824));
#28956=CARTESIAN_POINT('Ctrl Pts',(40.5730966676381,-74.,-23.6633713879345));
#28957=CARTESIAN_POINT('Ctrl Pts',(40.699999999979,-74.,-23.4706975310694));
#28958=CARTESIAN_POINT('Ctrl Pts',(40.4380952380952,-73.8333333333333,-24.1239304942116));
#28959=CARTESIAN_POINT('Ctrl Pts',(40.5728443653613,-73.8333333333333,-23.9527761154313));
#28960=CARTESIAN_POINT('Ctrl Pts',(40.7003137824798,-73.8269970069562,-23.7726894470159));
#28961=CARTESIAN_POINT('Ctrl Pts',(40.8245617157746,-73.8157835059031,-23.5830861153787));
#28962=CARTESIAN_POINT('Ctrl Pts',(40.5690476190476,-73.6666666666667,-24.2270287565669));
#28963=CARTESIAN_POINT('Ctrl Pts',(40.7010262035101,-73.6666666666667,-24.0593934397802));
#28964=CARTESIAN_POINT('Ctrl Pts',(40.8275308973216,-73.6539940139125,-23.8820075060973));
#28965=CARTESIAN_POINT('Ctrl Pts',(40.9491234315702,-73.6315670118063,-23.695474699688));
#28966=CARTESIAN_POINT('Ctrl Pts',(40.7,-73.5,-24.3301270189222));
#28967=CARTESIAN_POINT('Ctrl Pts',(40.8292080416589,-73.5,-24.1660107641291));
#28968=CARTESIAN_POINT('Ctrl Pts',(40.9547480121633,-73.4809910208687,-23.9913255651788));
#28969=CARTESIAN_POINT('Ctrl Pts',(41.0736851473658,-73.4473505177094,-23.8078632839972));
#28970=CARTESIAN_POINT('Origin',(40.7,-72.5,-10.));
#28971=CARTESIAN_POINT('',(42.1309672031646,-72.9498142544064,19.7928705636776));
#28972=CARTESIAN_POINT('Ctrl Pts',(42.1309672031646,-72.9498142544064,19.7928705636776));
#28973=CARTESIAN_POINT('Ctrl Pts',(42.1313015191887,-72.9487507148203,19.7904622190261));
#28974=CARTESIAN_POINT('Ctrl Pts',(42.131635265947,-72.9476850562422,19.7880498434514));
#28975=CARTESIAN_POINT('Ctrl Pts',(42.1319930273681,-72.9465377582794,19.7854527089951));
#28976=CARTESIAN_POINT('Ctrl Pts',(42.1323595522132,-72.9453623570669,19.7827919573092));
#28977=CARTESIAN_POINT('Ctrl Pts',(42.1327512677083,-72.9441013224905,19.7799374088966));
#28978=CARTESIAN_POINT('Ctrl Pts',(42.1331869934536,-72.9426906841072,19.7767444396953));
#28979=CARTESIAN_POINT('Ctrl Pts',(42.1336348579266,-72.9412407472539,19.7734625187076));
#28980=CARTESIAN_POINT('Ctrl Pts',(42.1341292064887,-72.9396328187942,19.7698232013363));
#28981=CARTESIAN_POINT('Ctrl Pts',(42.1346827212214,-72.9378190144668,19.7657193064195));
#28982=CARTESIAN_POINT('Ctrl Pts',(42.1352541149661,-72.935946622667,19.7614828520934));
#28983=CARTESIAN_POINT('Ctrl Pts',(42.1358885383903,-72.9338549128763,19.7567514907766));
#28984=CARTESIAN_POINT('Ctrl Pts',(42.1365920268532,-72.9315128600421,19.7514573859948));
#28985=CARTESIAN_POINT('Ctrl Pts',(42.1373390290756,-72.9290259412592,19.7458358182707));
#28986=CARTESIAN_POINT('Ctrl Pts',(42.1381638928087,-72.9262567586801,19.7395797654784));
#28987=CARTESIAN_POINT('Ctrl Pts',(42.1390652414578,-72.9231917187612,19.7326623902347));
#28988=CARTESIAN_POINT('Ctrl Pts',(42.140014214902,-72.9199647305237,19.7253795198202));
#28989=CARTESIAN_POINT('Ctrl Pts',(42.141047895993,-72.9164098916718,19.7173638532995));
#28990=CARTESIAN_POINT('Ctrl Pts',(42.1421560896575,-72.9125358324603,19.7086402766379));
#28991=CARTESIAN_POINT('Ctrl Pts',(42.1433432444181,-72.9083857384985,19.6992951270539));
#28992=CARTESIAN_POINT('Ctrl Pts',(42.144615779129,-72.9038694395542,19.6891379478677));
#28993=CARTESIAN_POINT('Ctrl Pts',(42.1459531129161,-72.8990233016358,19.6782576409165));
#28994=CARTESIAN_POINT('Ctrl Pts',(42.1474361260665,-72.8936492608903,19.6661921128894));
#28995=CARTESIAN_POINT('Ctrl Pts',(42.1489985826526,-72.8878698046632,19.653237905392));
#28996=CARTESIAN_POINT('Ctrl Pts',(42.1506057775466,-72.8817628559047,19.6395787815669));
#28997=CARTESIAN_POINT('Ctrl Pts',(42.1525799655489,-72.8742614228087,19.6228006804931));
#28998=CARTESIAN_POINT('Ctrl Pts',(42.1546209561383,-72.8662663804073,19.6049605042071));
#28999=CARTESIAN_POINT('Ctrl Pts',(42.1566625052706,-72.8579585810379,19.5864748262644));
#29000=CARTESIAN_POINT('Ctrl Pts',(42.1587486638376,-72.849469249798,19.567585221897));
#29001=CARTESIAN_POINT('Ctrl Pts',(42.1608345516525,-72.840655794778,19.5480271658165));
#29002=CARTESIAN_POINT('Ctrl Pts',(42.1628608842072,-72.831719811673,19.5282555859895));
#29003=CARTESIAN_POINT('Ctrl Pts',(42.1644778474499,-72.8245891182514,19.5124783544806));
#29004=CARTESIAN_POINT('Ctrl Pts',(42.1660570689819,-72.8173810964839,19.4965664787151));
#29005=CARTESIAN_POINT('Ctrl Pts',(42.1675779259144,-72.8101854789778,19.4807189369477));
#29006=CARTESIAN_POINT('Ctrl Pts',(42.1689362597088,-72.8037588058168,19.4665649089913));
#29007=CARTESIAN_POINT('Ctrl Pts',(42.1702481373004,-72.797342287202,19.4524626884228));
#29008=CARTESIAN_POINT('Ctrl Pts',(42.1715056420027,-72.7909830674702,19.438514996399));
#29009=CARTESIAN_POINT('Ctrl Pts',(42.1726775405847,-72.7850567591446,19.4255168100099));
#29010=CARTESIAN_POINT('Ctrl Pts',(42.1738022893872,-72.7791803848424,19.4126531571166));
#29011=CARTESIAN_POINT('Ctrl Pts',(42.1748785703465,-72.7733737418493,19.3999657009192));
#29012=CARTESIAN_POINT('Ctrl Pts',(42.1759006966771,-72.767859268473,19.3879166323786));
#29013=CARTESIAN_POINT('Ctrl Pts',(42.1768791687987,-72.7624078121534,19.3760267222246));
#29014=CARTESIAN_POINT('Ctrl Pts',(42.1778167095488,-72.7570170674844,19.3642888110875));
#29015=CARTESIAN_POINT('Ctrl Pts',(42.1787167504197,-72.7518419425355,19.3530203944763));
#29016=CARTESIAN_POINT('Ctrl Pts',(42.1795791195132,-72.7467228693616,19.3418922583279));
#29017=CARTESIAN_POINT('Ctrl Pts',(42.1804090975907,-72.7416379601195,19.33085433272));
#29018=CARTESIAN_POINT('Ctrl Pts',(42.1812615514281,-72.7364153518196,19.3195175007041));
#29019=CARTESIAN_POINT('Ctrl Pts',(42.1820798756141,-72.7312290975577,19.3082765013242));
#29020=CARTESIAN_POINT('Ctrl Pts',(42.1828722837951,-72.726030506685,19.2970223926875));
#29021=CARTESIAN_POINT('Ctrl Pts',(42.1836281590859,-72.7210715897002,19.2862871392632));
#29022=CARTESIAN_POINT('Ctrl Pts',(42.1843609603366,-72.7160979024093,19.2755321772426));
#29023=CARTESIAN_POINT('Ctrl Pts',(42.1850752052954,-72.7110725813951,19.2646751321278));
#29024=CARTESIAN_POINT('Ctrl Pts',(42.1858149431324,-72.7058678962916,19.2534305766423));
#29025=CARTESIAN_POINT('Ctrl Pts',(42.1865346966888,-72.7006079027222,19.242076712873));
#29026=CARTESIAN_POINT('Ctrl Pts',(42.1872349687888,-72.6952745441982,19.2305723771825));
#29027=CARTESIAN_POINT('Ctrl Pts',(42.1879839033092,-72.6895705666895,19.2182685967903));
#29028=CARTESIAN_POINT('Ctrl Pts',(42.188710468047,-72.6837826832338,19.2057927504724));
#29029=CARTESIAN_POINT('Ctrl Pts',(42.1894114918279,-72.6779140466942,19.1931496070932));
#29030=CARTESIAN_POINT('Ctrl Pts',(42.1901552158863,-72.6716879438093,19.1797363532756));
#29031=CARTESIAN_POINT('Ctrl Pts',(42.1908700606504,-72.6653710903413,19.1661351289144));
#29032=CARTESIAN_POINT('Ctrl Pts',(42.1915498829022,-72.6589935433102,19.1524086586535));
#29033=CARTESIAN_POINT('Ctrl Pts',(42.1922885178562,-72.6520642626857,19.137494685623));
#29034=CARTESIAN_POINT('Ctrl Pts',(42.1929856231885,-72.6450635503653,19.1224333500704));
#29035=CARTESIAN_POINT('Ctrl Pts',(42.1936332007538,-72.6380574576258,19.1073643725427));
#29036=CARTESIAN_POINT('Ctrl Pts',(42.1943843319655,-72.629931025811,19.0898857260347));
#29037=CARTESIAN_POINT('Ctrl Pts',(42.1950684825543,-72.6217977758197,19.0723977124727));
#29038=CARTESIAN_POINT('Ctrl Pts',(42.1956775765982,-72.6137918576236,19.0551850276049));
#29039=CARTESIAN_POINT('Ctrl Pts',(42.1964581307011,-72.6035322723288,19.0331269695248));
#29040=CARTESIAN_POINT('Ctrl Pts',(42.1971144713312,-72.5934842851803,19.0115263308462));
#29041=CARTESIAN_POINT('Ctrl Pts',(42.1976485567532,-72.5839571346295,18.9910403059571));
#29042=CARTESIAN_POINT('Ctrl Pts',(42.1980302734834,-72.5771479752563,18.9763987184592));
#29043=CARTESIAN_POINT('Ctrl Pts',(42.1983500908979,-72.5706057773694,18.9623284423976));
#29044=CARTESIAN_POINT('Ctrl Pts',(42.198615480378,-72.5644332365437,18.9490480914424));
#29045=CARTESIAN_POINT('Ctrl Pts',(42.1988537012205,-72.558892595386,18.9371272858667));
#29046=CARTESIAN_POINT('Ctrl Pts',(42.1990482194242,-72.5536501237203,18.9258436467134));
#29047=CARTESIAN_POINT('Ctrl Pts',(42.1992071494618,-72.5487639518768,18.9153211961306));
#29048=CARTESIAN_POINT('Ctrl Pts',(42.1993555433282,-72.5442017058562,18.9054963250792));
#29049=CARTESIAN_POINT('Ctrl Pts',(42.1994730023575,-72.5399502842729,18.8963354981348));
#29050=CARTESIAN_POINT('Ctrl Pts',(42.1995670103066,-72.5360386126285,18.8879006581744));
#29051=CARTESIAN_POINT('Ctrl Pts',(42.1996563826467,-72.5323198287168,18.8798817470811));
#29052=CARTESIAN_POINT('Ctrl Pts',(42.1997246147537,-72.5289082579991,18.8725193063125));
#29053=CARTESIAN_POINT('Ctrl Pts',(42.1997779466118,-72.5258091235177,18.8658247656506));
#29054=CARTESIAN_POINT('Ctrl Pts',(42.1998291813324,-72.5228318544961,18.859393470511));
#29055=CARTESIAN_POINT('Ctrl Pts',(42.1998666928339,-72.5201430455938,18.8535788292267));
#29056=CARTESIAN_POINT('Ctrl Pts',(42.1998952486401,-72.5177269034724,18.8483473578671));
#29057=CARTESIAN_POINT('Ctrl Pts',(42.1999224505203,-72.5154253187169,18.8433639280339));
#29058=CARTESIAN_POINT('Ctrl Pts',(42.1999415314425,-72.5133711925042,18.8389097594422));
#29059=CARTESIAN_POINT('Ctrl Pts',(42.1999556780803,-72.5115309927879,18.8349133527288));
#29060=CARTESIAN_POINT('Ctrl Pts',(42.1999695051995,-72.5097323561677,18.8310072096074));
#29061=CARTESIAN_POINT('Ctrl Pts',(42.1999786158394,-72.5081381842292,18.8275385861549));
#29062=CARTESIAN_POINT('Ctrl Pts',(42.199985051483,-72.5066966654099,18.824396763848));
#29063=CARTESIAN_POINT('Ctrl Pts',(42.1999912849262,-72.5053004374158,18.8213536539011));
#29064=CARTESIAN_POINT('Ctrl Pts',(42.1999950012483,-72.5040474594342,18.8186172174944));
#29065=CARTESIAN_POINT('Ctrl Pts',(42.1999972537806,-72.5028703049579,18.8160431766832));
#29066=CARTESIAN_POINT('Ctrl Pts',(42.1999991536502,-72.5018774490895,18.8138721349243));
#29067=CARTESIAN_POINT('Ctrl Pts',(42.2,-72.5009382344174,18.8118159788019));
#29068=CARTESIAN_POINT('Ctrl Pts',(42.2,-72.5,18.8097619285762));
#29069=CARTESIAN_POINT('Ctrl Pts',(40.699999999979,-74.,23.4706975310694));
#29070=CARTESIAN_POINT('Ctrl Pts',(41.0578917243185,-74.000000000005,22.9273203194824));
#29071=CARTESIAN_POINT('Ctrl Pts',(41.704007781412,-73.7466614991037,21.7070010142552));
#29072=CARTESIAN_POINT('Ctrl Pts',(42.0459074091364,-73.2204098933174,20.4056240222309));
#29073=CARTESIAN_POINT('Ctrl Pts',(42.1309672031646,-72.9498142544064,19.7928705636776));
#29074=CARTESIAN_POINT('Ctrl Pts',(34.9928678625178,-72.9498130615485,26.9309675781304));
#29075=CARTESIAN_POINT('Ctrl Pts',(34.9859788311223,-72.9467708226893,26.9319238812613));
#29076=CARTESIAN_POINT('Ctrl Pts',(34.9715230299339,-72.9403539923989,26.9337971106498));
#29077=CARTESIAN_POINT('Ctrl Pts',(34.8878030652082,-72.9035139065405,26.945647981921));
#29078=CARTESIAN_POINT('Ctrl Pts',(34.6364938840975,-72.7907445312107,26.9734428466108));
#29079=CARTESIAN_POINT('Ctrl Pts',(34.3664430831556,-72.6655778826375,26.9924900108967));
#29080=CARTESIAN_POINT('Ctrl Pts',(34.115145417116,-72.548594380104,27.0001343922656));
#29081=CARTESIAN_POINT('Ctrl Pts',(34.0311909778797,-72.5097908317003,26.9998426440259));
#29082=CARTESIAN_POINT('Ctrl Pts',(34.0166823597247,-72.5031611812015,27.));
#29083=CARTESIAN_POINT('Ctrl Pts',(34.0097619285762,-72.5,27.));
#29084=CARTESIAN_POINT('Ctrl Pts',(35.1322262809334,-72.648770594606,26.9529186924328));
#29085=CARTESIAN_POINT('Ctrl Pts',(35.127125742256,-72.6464928862312,26.9533741257474));
#29086=CARTESIAN_POINT('Ctrl Pts',(35.1181028925982,-72.6424664124947,26.9541647811871));
#29087=CARTESIAN_POINT('Ctrl Pts',(35.0602284162512,-72.6172306769364,26.9623825500304));
#29088=CARTESIAN_POINT('Ctrl Pts',(34.8622816998021,-72.5287879873221,26.985106682172));
#29089=CARTESIAN_POINT('Ctrl Pts',(34.6764678135481,-72.4421788390646,26.9974829453611));
#29090=CARTESIAN_POINT('Ctrl Pts',(34.4786154337669,-72.349707994528,27.0015588663316));
#29091=CARTESIAN_POINT('Ctrl Pts',(34.4206366608306,-72.3228010801069,26.9999951100012));
#29092=CARTESIAN_POINT('Ctrl Pts',(34.4116122748509,-72.3186769260278,27.));
#29093=CARTESIAN_POINT('Ctrl Pts',(34.4065079523841,-72.3163422783269,27.));
#29094=CARTESIAN_POINT('Ctrl Pts',(35.271584699349,-72.3477281276635,26.9748698067351));
#29095=CARTESIAN_POINT('Ctrl Pts',(35.2683080889331,-72.346245599186,26.9750197376988));
#29096=CARTESIAN_POINT('Ctrl Pts',(35.259759695035,-72.3423622132382,26.9755923652128));
#29097=CARTESIAN_POINT('Ctrl Pts',(35.2158882710644,-72.3223171563717,26.978929412466));
#29098=CARTESIAN_POINT('Ctrl Pts',(35.1084432567777,-72.2729880991628,26.9857191223274));
#29099=CARTESIAN_POINT('Ctrl Pts',(34.9662743319328,-72.2076840197809,26.9947085888439));
#29100=CARTESIAN_POINT('Ctrl Pts',(34.8589743510709,-72.1582939366101,26.9983926839512));
#29101=CARTESIAN_POINT('Ctrl Pts',(34.8151072057806,-72.1381226350592,26.9997583651705));
#29102=CARTESIAN_POINT('Ctrl Pts',(34.8065421899769,-72.1341926708542,27.));
#29103=CARTESIAN_POINT('Ctrl Pts',(34.8032539761921,-72.1326845566538,27.));
#29104=CARTESIAN_POINT('Ctrl Pts',(35.4109431177646,-72.046685660721,26.9968209210375));
#29105=CARTESIAN_POINT('Ctrl Pts',(35.4094718360417,-72.0460042802042,26.9968652778614));
#29106=CARTESIAN_POINT('Ctrl Pts',(35.4063833562612,-72.0445740141917,26.996951976694));
#29107=CARTESIAN_POINT('Ctrl Pts',(35.3884438670994,-72.0362655625548,26.9975052710777));
#29108=CARTESIAN_POINT('Ctrl Pts',(35.3344712811044,-72.0112736209447,26.9987929427077));
#29109=CARTESIAN_POINT('Ctrl Pts',(35.2764806026585,-71.9844299049754,26.9996557904983));
#29110=CARTESIAN_POINT('Ctrl Pts',(35.2225217556451,-71.9594531196762,27.0000060026486));
#29111=CARTESIAN_POINT('Ctrl Pts',(35.2045600360351,-71.9511381093811,26.9999927641665));
#29112=CARTESIAN_POINT('Ctrl Pts',(35.2014721051031,-71.9497084156806,27.));
#29113=CARTESIAN_POINT('Ctrl Pts',(35.2,-71.9490268349807,27.));
#29114=CARTESIAN_POINT('',(34.0097619285762,-72.5,27.));
#29115=CARTESIAN_POINT('',(34.9928678625178,-72.9498130615485,26.9309675781304));
#29116=CARTESIAN_POINT('Ctrl Pts',(34.0097619285762,-72.5,27.));
#29117=CARTESIAN_POINT('Ctrl Pts',(34.0121798317656,-72.5011044731095,27.));
#29118=CARTESIAN_POINT('Ctrl Pts',(34.0146017561988,-72.5022108180881,26.9999988447398));
#29119=CARTESIAN_POINT('Ctrl Pts',(34.0172080806341,-72.5034032651581,26.9999961392571));
#29120=CARTESIAN_POINT('Ctrl Pts',(34.0198781898187,-72.5046248950636,26.999993367563));
#29121=CARTESIAN_POINT('Ctrl Pts',(34.0227417110302,-72.5059368360811,26.9999889713356));
#29122=CARTESIAN_POINT('Ctrl Pts',(34.0259430017054,-72.5074065633977,26.9999817141614));
#29123=CARTESIAN_POINT('Ctrl Pts',(34.0292333827049,-72.5089171924931,26.9999742550237));
#29124=CARTESIAN_POINT('Ctrl Pts',(34.0328804521166,-72.5105944472574,26.9999637812448));
#29125=CARTESIAN_POINT('Ctrl Pts',(34.0369912120385,-72.5124884140809,26.9999480122703));
#29126=CARTESIAN_POINT('Ctrl Pts',(34.0412345913922,-72.5144434831844,26.9999317345645));
#29127=CARTESIAN_POINT('Ctrl Pts',(34.0459718952787,-72.5166293969508,26.9999098171331));
#29128=CARTESIAN_POINT('Ctrl Pts',(34.0512708767212,-72.5190779485735,26.999878672386));
#29129=CARTESIAN_POINT('Ctrl Pts',(34.0568972279557,-72.5216777711233,26.9998456035239));
#29130=CARTESIAN_POINT('Ctrl Pts',(34.0631567735687,-72.5245736760052,26.9998021229674));
#29131=CARTESIAN_POINT('Ctrl Pts',(34.070076378992,-72.5277783735895,26.9997427652637));
#29132=CARTESIAN_POINT('Ctrl Pts',(34.0773609213403,-72.531152085505,26.9996802770609));
#29133=CARTESIAN_POINT('Ctrl Pts',(34.0853767252336,-72.5348679050113,26.9996001514933));
#29134=CARTESIAN_POINT('Ctrl Pts',(34.0940990871599,-72.5389144011236,26.9994951381666));
#29135=CARTESIAN_POINT('Ctrl Pts',(34.1034413765545,-72.5432484952639,26.9993826611911));
#29136=CARTESIAN_POINT('Ctrl Pts',(34.1135938746767,-72.5479617814953,26.9992415459466));
#29137=CARTESIAN_POINT('Ctrl Pts',(34.1244680994071,-72.5530128872092,26.999062918556));
#29138=CARTESIAN_POINT('Ctrl Pts',(34.1365221810635,-72.5586120395387,26.9988649100354));
#29139=CARTESIAN_POINT('Ctrl Pts',(34.1494625299636,-72.5646260341558,26.9986206326567));
#29140=CARTESIAN_POINT('Ctrl Pts',(34.163106332895,-72.5709691128917,26.9983201877487));
#29141=CARTESIAN_POINT('Ctrl Pts',(34.1798085686584,-72.578734073808,26.9979523942742));
#29142=CARTESIAN_POINT('Ctrl Pts',(34.1975634699253,-72.5869914895447,26.997499916619));
#29143=CARTESIAN_POINT('Ctrl Pts',(34.2159606405676,-72.5955484292679,26.9969537393201));
#29144=CARTESIAN_POINT('Ctrl Pts',(34.2348611311504,-72.6043394744671,26.9963926194015));
#29145=CARTESIAN_POINT('Ctrl Pts',(34.2544339880504,-72.6134440505946,26.9957325028427));
#29146=CARTESIAN_POINT('Ctrl Pts',(34.2742231414687,-72.6226474512814,26.9949774589251));
#29147=CARTESIAN_POINT('Ctrl Pts',(34.2900236652418,-72.6299958480658,26.9943745989079));
#29148=CARTESIAN_POINT('Ctrl Pts',(34.3059607360667,-72.6374066137588,26.993711612265));
#29149=CARTESIAN_POINT('Ctrl Pts',(34.3218342018758,-72.644785372866,26.9929960468146));
#29150=CARTESIAN_POINT('Ctrl Pts',(34.3360016106727,-72.6513710736792,26.9923573892978));
#29151=CARTESIAN_POINT('Ctrl Pts',(34.3501178623903,-72.6579310555955,26.9916770268009));
#29152=CARTESIAN_POINT('Ctrl Pts',(34.3640796025327,-72.6644163574706,26.9909618577939));
#29153=CARTESIAN_POINT('Ctrl Pts',(34.3770874324976,-72.6704585630411,26.9902955513919));
#29154=CARTESIAN_POINT('Ctrl Pts',(34.389960814589,-72.6764358005933,26.9895991550423));
#29155=CARTESIAN_POINT('Ctrl Pts',(34.4026575542914,-72.6823276467199,26.9888776407891));
#29156=CARTESIAN_POINT('Ctrl Pts',(34.4147137119833,-72.6879222345956,26.9881925287195));
#29157=CARTESIAN_POINT('Ctrl Pts',(34.4266103549825,-72.6934397254313,26.9874848652868));
#29158=CARTESIAN_POINT('Ctrl Pts',(34.4383541181474,-72.6988823143506,26.9867568143575));
#29159=CARTESIAN_POINT('Ctrl Pts',(34.4496271379255,-72.7041067395769,26.9860579470175));
#29160=CARTESIAN_POINT('Ctrl Pts',(34.4607590909511,-72.7092620662248,26.9853403733255));
#29161=CARTESIAN_POINT('Ctrl Pts',(34.4717994954728,-72.7143701921677,26.9846027821306));
#29162=CARTESIAN_POINT('Ctrl Pts',(34.4830516132264,-72.7195762726604,26.9838510467243));
#29163=CARTESIAN_POINT('Ctrl Pts',(34.494208022994,-72.7247330573083,26.9830786440325));
#29164=CARTESIAN_POINT('Ctrl Pts',(34.5053743623492,-72.7298878885211,26.9822791770484));
#29165=CARTESIAN_POINT('Ctrl Pts',(34.5161068521514,-72.7348424373365,26.981510772025));
#29166=CARTESIAN_POINT('Ctrl Pts',(34.5268564287903,-72.7397987793137,26.9807167793456));
#29167=CARTESIAN_POINT('Ctrl Pts',(34.5377063841563,-72.7447940225827,26.9798904981477));
#29168=CARTESIAN_POINT('Ctrl Pts',(34.5489423003185,-72.7499669594922,26.9790348240041));
#29169=CARTESIAN_POINT('Ctrl Pts',(34.5602856719162,-72.7551815188518,26.9781444707592));
#29170=CARTESIAN_POINT('Ctrl Pts',(34.5717785652466,-72.7604559078742,26.9772145138921));
#29171=CARTESIAN_POINT('Ctrl Pts',(34.5840671780162,-72.766095473337,26.9762201707355));
#29172=CARTESIAN_POINT('Ctrl Pts',(34.5965266886173,-72.7718034060858,26.9751804717666));
#29173=CARTESIAN_POINT('Ctrl Pts',(34.6091533215573,-72.7775769562531,26.974093291945));
#29174=CARTESIAN_POINT('Ctrl Pts',(34.6225448421687,-72.7837002526563,26.9729402536759));
#29175=CARTESIAN_POINT('Ctrl Pts',(34.6361240193327,-72.789897187906,26.9717337257247));
#29176=CARTESIAN_POINT('Ctrl Pts',(34.649829260066,-72.7961388946458,26.9704767101447));
#29177=CARTESIAN_POINT('Ctrl Pts',(34.6647111637454,-72.8029164828914,26.9691117735377));
#29178=CARTESIAN_POINT('Ctrl Pts',(34.6797412183778,-72.8097466039824,26.967687199764));
#29179=CARTESIAN_POINT('Ctrl Pts',(34.6947812708973,-72.8165662126057,26.9662147977143));
#29180=CARTESIAN_POINT('Ctrl Pts',(34.7121784708218,-72.8244546222023,26.9645116339259));
#29181=CARTESIAN_POINT('Ctrl Pts',(34.7295881416525,-72.83232847794,26.9627442813414));
#29182=CARTESIAN_POINT('Ctrl Pts',(34.7467301342148,-72.8400621253298,26.9609441299777));
#29183=CARTESIAN_POINT('Ctrl Pts',(34.7690864666648,-72.8501482335504,26.9585963992689));
#29184=CARTESIAN_POINT('Ctrl Pts',(34.7909822100655,-72.8599932152628,26.9561926445279));
#29185=CARTESIAN_POINT('Ctrl Pts',(34.8117335912673,-72.8692963615804,26.9538294938965));
#29186=CARTESIAN_POINT('Ctrl Pts',(34.8263877334338,-72.8758660268672,26.9521606919515));
#29187=CARTESIAN_POINT('Ctrl Pts',(34.8404692081152,-72.8821647678184,26.9505129508526));
#29188=CARTESIAN_POINT('Ctrl Pts',(34.8537584983512,-72.8880981139686,26.9489236880989));
#29189=CARTESIAN_POINT('Ctrl Pts',(34.8656824913596,-72.8934218879817,26.9474977008846));
#29190=CARTESIAN_POINT('Ctrl Pts',(34.8769680122958,-72.8984512256775,26.9461190319871));
#29191=CARTESIAN_POINT('Ctrl Pts',(34.8874906704523,-72.9031338368634,26.9448124824959));
#29192=CARTESIAN_POINT('Ctrl Pts',(34.8973142788575,-72.9075053690295,26.9435927307589));
#29193=CARTESIAN_POINT('Ctrl Pts',(34.9064725793694,-72.9115745492444,26.9424359792807));
#29194=CARTESIAN_POINT('Ctrl Pts',(34.9149034806463,-72.9153163971448,26.9413577939785));
#29195=CARTESIAN_POINT('Ctrl Pts',(34.9229180225557,-72.9188734541938,26.940332854769));
#29196=CARTESIAN_POINT('Ctrl Pts',(34.9302749193298,-72.9221345908904,26.9393790077743));
#29197=CARTESIAN_POINT('Ctrl Pts',(34.9369627380912,-72.9250967827356,26.9385036410478));
#29198=CARTESIAN_POINT('Ctrl Pts',(34.9433872602677,-72.9279423543456,26.9376627371377));
#29199=CARTESIAN_POINT('Ctrl Pts',(34.9491941014795,-72.9305119583031,26.9368943156628));
#29200=CARTESIAN_POINT('Ctrl Pts',(34.9544168588578,-72.9328219368754,26.9361981656302));
#29201=CARTESIAN_POINT('Ctrl Pts',(34.9593918014892,-72.9350223092159,26.9355350472381));
#29202=CARTESIAN_POINT('Ctrl Pts',(34.9638366931368,-72.9369870780134,26.9349375205311));
#29203=CARTESIAN_POINT('Ctrl Pts',(34.9678232367822,-72.9387488347673,26.9343986405426));
#29204=CARTESIAN_POINT('Ctrl Pts',(34.9717196612948,-72.9404707655454,26.9338719423841));
#29205=CARTESIAN_POINT('Ctrl Pts',(34.9751780232743,-72.941998670718,26.933401294822));
#29206=CARTESIAN_POINT('Ctrl Pts',(34.9783093387544,-72.9433820368175,26.9329732619374));
#29207=CARTESIAN_POINT('Ctrl Pts',(34.9813422498734,-72.9447219294127,26.9325586803651));
#29208=CARTESIAN_POINT('Ctrl Pts',(34.9840682614716,-72.9459261859505,26.9321840818727));
#29209=CARTESIAN_POINT('Ctrl Pts',(34.9866320307011,-72.9470587250239,26.9318304705446));
#29210=CARTESIAN_POINT('Ctrl Pts',(34.988787344238,-72.9480108297485,26.9315331960187));
#29211=CARTESIAN_POINT('Ctrl Pts',(34.9908286451645,-72.9489125305568,26.9312506527497));
#29212=CARTESIAN_POINT('Ctrl Pts',(34.9928678625178,-72.9498130615485,26.9309675781304));
#29213=CARTESIAN_POINT('Ctrl Pts',(35.4109431177646,-72.046685660721,26.9968209210375));
#29214=CARTESIAN_POINT('Ctrl Pts',(35.271584699349,-72.3477281276635,26.9748698067351));
#29215=CARTESIAN_POINT('Ctrl Pts',(35.1322262809334,-72.648770594606,26.9529186924328));
#29216=CARTESIAN_POINT('Ctrl Pts',(34.9928678625178,-72.9498130615485,26.9309675781304));
#29217=CARTESIAN_POINT('',(34.6048809642881,-72.2245134174903,27.));
#29218=CARTESIAN_POINT('Ctrl Pts',(42.196820839876,-72.0466869074717,20.2109458098101));
#29219=CARTESIAN_POINT('Ctrl Pts',(42.1968651977585,-72.0460055194057,20.2094745117698));
#29220=CARTESIAN_POINT('Ctrl Pts',(42.1969518986639,-72.0445752373298,20.2063859972174));
#29221=CARTESIAN_POINT('Ctrl Pts',(42.1975052069546,-72.0362666836179,20.1884462883035));
#29222=CARTESIAN_POINT('Ctrl Pts',(42.1987929121607,-72.0112744135499,20.1344729899145));
#29223=CARTESIAN_POINT('Ctrl Pts',(42.1996557821269,-71.9844303509257,20.0764815416121));
#29224=CARTESIAN_POINT('Ctrl Pts',(42.2000060028006,-71.9594532548772,20.022522027641));
#29225=CARTESIAN_POINT('Ctrl Pts',(42.1999927639906,-71.9511381376986,20.004560090378));
#29226=CARTESIAN_POINT('Ctrl Pts',(42.2,-71.9497084248624,20.0014721226316));
#29227=CARTESIAN_POINT('Ctrl Pts',(42.2,-71.9490268349807,20.));
#29228=CARTESIAN_POINT('Ctrl Pts',(42.1748696276389,-72.3477293564499,20.0715873944326));
#29229=CARTESIAN_POINT('Ctrl Pts',(42.1750195593748,-72.3462468301403,20.0683107887067));
#29230=CARTESIAN_POINT('Ctrl Pts',(42.1755112872819,-72.342363439581,20.0597605016236));
#29231=CARTESIAN_POINT('Ctrl Pts',(42.1782699776807,-72.3223182757032,20.0159145750237));
#29232=CARTESIAN_POINT('Ctrl Pts',(42.1845158453337,-72.2729887945663,19.9085740298018));
#29233=CARTESIAN_POINT('Ctrl Pts',(42.1930982717819,-72.207684249358,19.7663902797076));
#29234=CARTESIAN_POINT('Ctrl Pts',(42.1980895940111,-72.1582938438831,19.6590311049478));
#29235=CARTESIAN_POINT('Ctrl Pts',(42.1997838820197,-72.1381225623237,19.6151120158836));
#29236=CARTESIAN_POINT('Ctrl Pts',(42.2,-72.1341926423635,19.6065422105412));
#29237=CARTESIAN_POINT('Ctrl Pts',(42.2,-72.1326845566538,19.6032539761921));
#29238=CARTESIAN_POINT('Ctrl Pts',(42.1529184154018,-72.6487718054281,19.9322289790551));
#29239=CARTESIAN_POINT('Ctrl Pts',(42.1533738444073,-72.6464941085306,19.9271284658077));
#29240=CARTESIAN_POINT('Ctrl Pts',(42.1544898154414,-72.6425808645548,19.9181056666025));
#29241=CARTESIAN_POINT('Ctrl Pts',(42.162296347732,-72.6159506839129,19.8602311090506));
#29242=CARTESIAN_POINT('Ctrl Pts',(42.1782299355538,-72.5231682072857,19.6622832801377));
#29243=CARTESIAN_POINT('Ctrl Pts',(42.1937530235431,-72.4384015430389,19.4764686505132));
#29244=CARTESIAN_POINT('Ctrl Pts',(42.1979624296397,-72.3480974306778,19.2786157337193));
#29245=CARTESIAN_POINT('Ctrl Pts',(42.1994067391489,-72.3226741649949,19.2206367291843));
#29246=CARTESIAN_POINT('Ctrl Pts',(42.2,-72.3186768598647,19.2116122984507));
#29247=CARTESIAN_POINT('Ctrl Pts',(42.2,-72.3163422783269,19.2065079523841));
#29248=CARTESIAN_POINT('Ctrl Pts',(42.1309672031646,-72.9498142544064,19.7928705636776));
#29249=CARTESIAN_POINT('Ctrl Pts',(42.1319235023647,-72.9467720369169,19.7859815787116));
#29250=CARTESIAN_POINT('Ctrl Pts',(42.1337967255951,-72.9403552446875,19.7715258643937));
#29251=CARTESIAN_POINT('Ctrl Pts',(42.145647611726,-72.9035152339706,19.6878058974393));
#29252=CARTESIAN_POINT('Ctrl Pts',(42.1734427243359,-72.7907453606573,19.4364956174772));
#29253=CARTESIAN_POINT('Ctrl Pts',(42.1924901231468,-72.6655771656199,19.1664440243787));
#29254=CARTESIAN_POINT('Ctrl Pts',(42.2001344088158,-72.5485935297578,18.9151457627271));
#29255=CARTESIAN_POINT('Ctrl Pts',(42.1998426456441,-72.5097905257285,18.8311910575127));
#29256=CARTESIAN_POINT('Ctrl Pts',(42.2,-72.5031610773659,18.8166823863602));
#29257=CARTESIAN_POINT('Ctrl Pts',(42.2,-72.5,18.8097619285762));
#29258=CARTESIAN_POINT('Ctrl Pts',(42.1309672031646,-72.9498142544064,19.7928705636776));
#29259=CARTESIAN_POINT('Ctrl Pts',(42.1529184154018,-72.6487718054281,19.9322289790551));
#29260=CARTESIAN_POINT('Ctrl Pts',(42.1748696276389,-72.3477293564499,20.0715873944326));
#29261=CARTESIAN_POINT('Ctrl Pts',(42.196820839876,-72.0466869074717,20.2109458098101));
#29262=CARTESIAN_POINT('Ctrl Pts',(42.1309672031646,-72.9498142544064,19.7928705636776));
#29263=CARTESIAN_POINT('Ctrl Pts',(42.0459074091364,-73.2204098933174,20.4056240222309));
#29264=CARTESIAN_POINT('Ctrl Pts',(41.704007781412,-73.7466614991037,21.7070010142552));
#29265=CARTESIAN_POINT('Ctrl Pts',(41.0578917243185,-74.000000000005,22.9273203194824));
#29266=CARTESIAN_POINT('Ctrl Pts',(40.699999999979,-74.,23.4706975310694));
#29267=CARTESIAN_POINT('Ctrl Pts',(42.1529184154018,-72.6487718054281,19.9322289790551));
#29268=CARTESIAN_POINT('Ctrl Pts',(42.0900566190563,-72.9237208747561,20.544894147307));
#29269=CARTESIAN_POINT('Ctrl Pts',(41.7929657367318,-73.4750045131386,21.8418272713667));
#29270=CARTESIAN_POINT('Ctrl Pts',(41.1749647057687,-73.7841592833289,23.0483683735484));
#29271=CARTESIAN_POINT('Ctrl Pts',(40.8245617157746,-73.8157835059031,23.5830861153787));
#29272=CARTESIAN_POINT('Ctrl Pts',(42.1748696276389,-72.3477293564499,20.0715873944326));
#29273=CARTESIAN_POINT('Ctrl Pts',(42.1342058289762,-72.6270318561947,20.6841642723831));
#29274=CARTESIAN_POINT('Ctrl Pts',(41.8819236920516,-73.2033475271735,21.9766535284783));
#29275=CARTESIAN_POINT('Ctrl Pts',(41.2920376872189,-73.5683185666529,23.1694164276145));
#29276=CARTESIAN_POINT('Ctrl Pts',(40.9491234315702,-73.6315670118063,23.6954746996879));
#29277=CARTESIAN_POINT('Ctrl Pts',(42.196820839876,-72.0466869074717,20.2109458098101));
#29278=CARTESIAN_POINT('Ctrl Pts',(42.1783550388962,-72.3303428376334,20.8234343974591));
#29279=CARTESIAN_POINT('Ctrl Pts',(41.9708816473713,-72.9316905412085,22.1114797855899));
#29280=CARTESIAN_POINT('Ctrl Pts',(41.409110668669,-73.3524778499768,23.2904644816805));
#29281=CARTESIAN_POINT('Ctrl Pts',(41.0736851473658,-73.4473505177094,23.8078632839972));
#29282=CARTESIAN_POINT('',(41.0736851473658,-73.4473505177094,23.8078632839972));
#29283=CARTESIAN_POINT('Origin',(35.2,-73.75,20.));
#29284=CARTESIAN_POINT('',(39.5301270189222,-73.5,25.5));
#29285=CARTESIAN_POINT('',(40.3071428571429,-74.,24.0208322318563));
#29286=CARTESIAN_POINT('Ctrl Pts',(40.699999999979,-74.,23.4706975310694));
#29287=CARTESIAN_POINT('Ctrl Pts',(40.5730966676381,-74.,23.6633713879345));
#29288=CARTESIAN_POINT('Ctrl Pts',(40.4446625272125,-74.,23.8461587910824));
#29289=CARTESIAN_POINT('Ctrl Pts',(40.3071428571429,-74.,24.0208322318563));
#29290=CARTESIAN_POINT('Ctrl Pts',(40.8245617157746,-73.8157835059031,23.5830861153787));
#29291=CARTESIAN_POINT('Ctrl Pts',(40.7003137824799,-73.8269970069562,23.7726894470159));
#29292=CARTESIAN_POINT('Ctrl Pts',(40.5728443653613,-73.8333333333333,23.9527761154313));
#29293=CARTESIAN_POINT('Ctrl Pts',(40.4380952380953,-73.8333333333333,24.1239304942116));
#29294=CARTESIAN_POINT('Ctrl Pts',(40.9491234315702,-73.6315670118063,23.6954746996879));
#29295=CARTESIAN_POINT('Ctrl Pts',(40.8275308973216,-73.6539940139125,23.8820075060973));
#29296=CARTESIAN_POINT('Ctrl Pts',(40.7010262035101,-73.6666666666667,24.0593934397802));
#29297=CARTESIAN_POINT('Ctrl Pts',(40.5690476190476,-73.6666666666667,24.2270287565669));
#29298=CARTESIAN_POINT('Ctrl Pts',(41.0736851473658,-73.4473505177094,23.8078632839972));
#29299=CARTESIAN_POINT('Ctrl Pts',(40.9547480121633,-73.4809910208687,23.9913255651787));
#29300=CARTESIAN_POINT('Ctrl Pts',(40.8292080416589,-73.5,24.1660107641291));
#29301=CARTESIAN_POINT('Ctrl Pts',(40.7,-73.5,24.3301270189222));
#29302=CARTESIAN_POINT('Ctrl Pts',(38.670697532745,-74.,25.4999999988754));
#29303=CARTESIAN_POINT('Ctrl Pts',(38.3480203762685,-74.0000000001593,25.7125291250959));
#29304=CARTESIAN_POINT('Ctrl Pts',(37.8159361986621,-73.9255312874326,26.0143563494905));
#29305=CARTESIAN_POINT('Ctrl Pts',(36.6753333677337,-73.6438750005303,26.5487153899226));
#29306=CARTESIAN_POINT('Ctrl Pts',(35.6787076842961,-73.2526841673963,26.8357625004906));
#29307=CARTESIAN_POINT('Ctrl Pts',(34.9928678625178,-72.9498130615485,26.9309675781304));
#29308=CARTESIAN_POINT('Ctrl Pts',(38.7830861170276,-73.8157835060006,25.6245617146941));
#29309=CARTESIAN_POINT('Ctrl Pts',(38.4655512687303,-73.7970038922842,25.8326437580241));
#29310=CARTESIAN_POINT('Ctrl Pts',(37.9402230267678,-73.6962906722935,26.1238795687314));
#29311=CARTESIAN_POINT('Ctrl Pts',(36.8104945847949,-73.3693647115943,26.6290704767058));
#29312=CARTESIAN_POINT('Ctrl Pts',(35.8179633331108,-72.956512531518,26.8825594092965));
#29313=CARTESIAN_POINT('Ctrl Pts',(35.1322262809334,-72.648770594606,26.9529186924328));
#29314=CARTESIAN_POINT('Ctrl Pts',(38.8954747013101,-73.6315670120013,25.7491234305128));
#29315=CARTESIAN_POINT('Ctrl Pts',(38.5830821611921,-73.5940077844089,25.9527583909524));
#29316=CARTESIAN_POINT('Ctrl Pts',(38.0645098548735,-73.4670500571544,26.2334027879723));
#29317=CARTESIAN_POINT('Ctrl Pts',(36.9456558018562,-73.0948544226583,26.7094255634889));
#29318=CARTESIAN_POINT('Ctrl Pts',(35.9572189819256,-72.6603408956398,26.9293563181024));
#29319=CARTESIAN_POINT('Ctrl Pts',(35.271584699349,-72.3477281276635,26.9748698067351));
#29320=CARTESIAN_POINT('Ctrl Pts',(39.0078632855927,-73.4473505180019,25.8736851463315));
#29321=CARTESIAN_POINT('Ctrl Pts',(38.7006130536539,-73.3910116765338,26.0728730238806));
#29322=CARTESIAN_POINT('Ctrl Pts',(38.1887966829792,-73.2378094420153,26.3429260072132));
#29323=CARTESIAN_POINT('Ctrl Pts',(37.0808170189174,-72.8203441337222,26.7897806502721));
#29324=CARTESIAN_POINT('Ctrl Pts',(36.0964746307403,-72.3641692597616,26.9761532269083));
#29325=CARTESIAN_POINT('Ctrl Pts',(35.4109431177646,-72.046685660721,26.9968209210375));
#29326=CARTESIAN_POINT('Ctrl Pts',(34.9928678625178,-72.9498130615485,26.9309675781304));
#29327=CARTESIAN_POINT('Ctrl Pts',(35.6787076842961,-73.2526841673963,26.8357625004906));
#29328=CARTESIAN_POINT('Ctrl Pts',(36.6753333677337,-73.6438750005303,26.5487153899226));
#29329=CARTESIAN_POINT('Ctrl Pts',(37.8159361986621,-73.9255312874326,26.0143563494905));
#29330=CARTESIAN_POINT('Ctrl Pts',(38.3480203762685,-74.0000000001593,25.7125291250959));
#29331=CARTESIAN_POINT('Ctrl Pts',(38.670697532745,-74.,25.4999999988754));
#29332=CARTESIAN_POINT('',(38.6706975330488,-74.,25.4999999993376));
#29333=CARTESIAN_POINT('Ctrl Pts',(39.2208322318563,-74.,25.1071428571429));
#29334=CARTESIAN_POINT('Ctrl Pts',(39.0524411521674,-74.,25.2397164505804));
#29335=CARTESIAN_POINT('Ctrl Pts',(38.8678098322883,-74.,25.3701733162485));
#29336=CARTESIAN_POINT('Ctrl Pts',(38.6706975327445,-74.,25.4999999988757));
#29337=CARTESIAN_POINT('Ctrl Pts',(39.3239304942116,-73.8333333333333,25.2380952380952));
#29338=CARTESIAN_POINT('Ctrl Pts',(39.1589319088021,-73.8333333333333,25.3679979349617));
#29339=CARTESIAN_POINT('Ctrl Pts',(38.9770571586008,-73.8272553216869,25.4974516009823));
#29340=CARTESIAN_POINT('Ctrl Pts',(38.7830861170271,-73.8157835060006,25.6245617146944));
#29341=CARTESIAN_POINT('Ctrl Pts',(39.4270287565669,-73.6666666666667,25.3690476190476));
#29342=CARTESIAN_POINT('Ctrl Pts',(39.2654226654369,-73.6666666666667,25.496279419343));
#29343=CARTESIAN_POINT('Ctrl Pts',(39.0863044849134,-73.6545106433737,25.6247298857161));
#29344=CARTESIAN_POINT('Ctrl Pts',(38.8954747013097,-73.6315670120012,25.7491234305131));
#29345=CARTESIAN_POINT('Ctrl Pts',(39.5301270189222,-73.5,25.5));
#29346=CARTESIAN_POINT('Ctrl Pts',(39.3719134220716,-73.5,25.6245609037243));
#29347=CARTESIAN_POINT('Ctrl Pts',(39.195551811226,-73.4817659650606,25.75200817045));
#29348=CARTESIAN_POINT('Ctrl Pts',(39.0078632855922,-73.4473505180018,25.8736851463318));
#29349=CARTESIAN_POINT('Origin',(25.2,-72.5,25.5));
#29350=CARTESIAN_POINT('',(25.2,-72.5,27.));
#29351=CARTESIAN_POINT('Origin',(35.2,-32.,27.));
#29352=CARTESIAN_POINT('Origin',(35.2,-72.,4.));
#29353=CARTESIAN_POINT('',(35.2,-72.,4.));
#29354=CARTESIAN_POINT('Origin',(28.2,-72.,3.99999999999999));
#29355=CARTESIAN_POINT('',(28.2,-72.,11.));
#29356=CARTESIAN_POINT('Origin',(2.2,-72.,11.));
#29357=CARTESIAN_POINT('',(2.2,-72.,11.));
#29358=CARTESIAN_POINT('Origin',(2.2,-72.,4.));
#29359=CARTESIAN_POINT('Origin',(-7.1,-32.,-4.));
#29360=CARTESIAN_POINT('',(-7.1,-32.,4.));
#29361=CARTESIAN_POINT('',(-7.1,-32.,-4.));
#29362=CARTESIAN_POINT('Origin',(2.20000000000001,-32.,-3.99999999999999));
#29363=CARTESIAN_POINT('',(2.2,-32.,-13.3));
#29364=CARTESIAN_POINT('Origin',(28.2,-32.,-13.3));
#29365=CARTESIAN_POINT('Origin',(2.2,-32.,3.99999999999999));
#32290=UNCERTAINTY_MEASURE_WITH_UNIT(LENGTH_MEASURE(0.01),#32310,
'DISTANCE_ACCURACY_VALUE',
'Maximum model space distance between geometric entities at asserted c
onnectivities');
#32293=UNCERTAINTY_MEASURE_WITH_UNIT(LENGTH_MEASURE(0.01),#32310,
'DISTANCE_ACCURACY_VALUE',
'Maximum model space distance between geometric entities at asserted c
onnectivities');
#32306=(
GEOMETRIC_REPRESENTATION_CONTEXT(3)
GLOBAL_UNCERTAINTY_ASSIGNED_CONTEXT((#32290))
GLOBAL_UNIT_ASSIGNED_CONTEXT((#32310,#32312,#32313))
REPRESENTATION_CONTEXT('','3D')
);
#32309=(
GEOMETRIC_REPRESENTATION_CONTEXT(3)
GLOBAL_UNCERTAINTY_ASSIGNED_CONTEXT((#32293))
GLOBAL_UNIT_ASSIGNED_CONTEXT((#32310,#32312,#32313))
REPRESENTATION_CONTEXT('','3D')
);
#32310=(
LENGTH_UNIT()
NAMED_UNIT(*)
SI_UNIT(.MILLI.,.METRE.)
);
#32312=(
NAMED_UNIT(*)
PLANE_ANGLE_UNIT()
SI_UNIT($,.RADIAN.)
);
#32313=(
NAMED_UNIT(*)
SI_UNIT($,.STERADIAN.)
SOLID_ANGLE_UNIT()
);
#32326=SHAPE_DEFINITION_REPRESENTATION(#32341,#32373);
#32341=PRODUCT_DEFINITION_SHAPE('',$,#32389);
#32373=SHAPE_REPRESENTATION('',(#14690),#32306);
#32376=PRODUCT_DEFINITION_CONTEXT('part definition',#32423,'design');
#32389=PRODUCT_DEFINITION('2026-10-25-00-35-21-990',
'13_Rubber_Lock_Boot',#32404,#32376);
#32404=PRODUCT_DEFINITION_FORMATION('',$,#32437);
#32423=APPLICATION_CONTEXT(
'Core Data for Automotive Mechanical Design Process');
#32424=PRODUCT_CONTEXT('part definition',#32423,'mechanical');
#32437=PRODUCT('2026-10-25-00-35-21-990','13_Rubber_Lock_Boot',$,(#32424));
#32503=COLOUR_RGB('Black',0.12,0.14,0.17);
#32504=FILL_AREA_STYLE_COLOUR('',#32503);
#32505=FILL_AREA_STYLE('',(#32504));
#32506=SURFACE_STYLE_FILL_AREA(#32505);
#32507=SURFACE_SIDE_STYLE('',(#32506));
#32508=SURFACE_STYLE_USAGE(.BOTH.,#32507);
#32509=PRESENTATION_STYLE_ASSIGNMENT((#32508));
ENDSEC;
END-ISO-10303-21;
